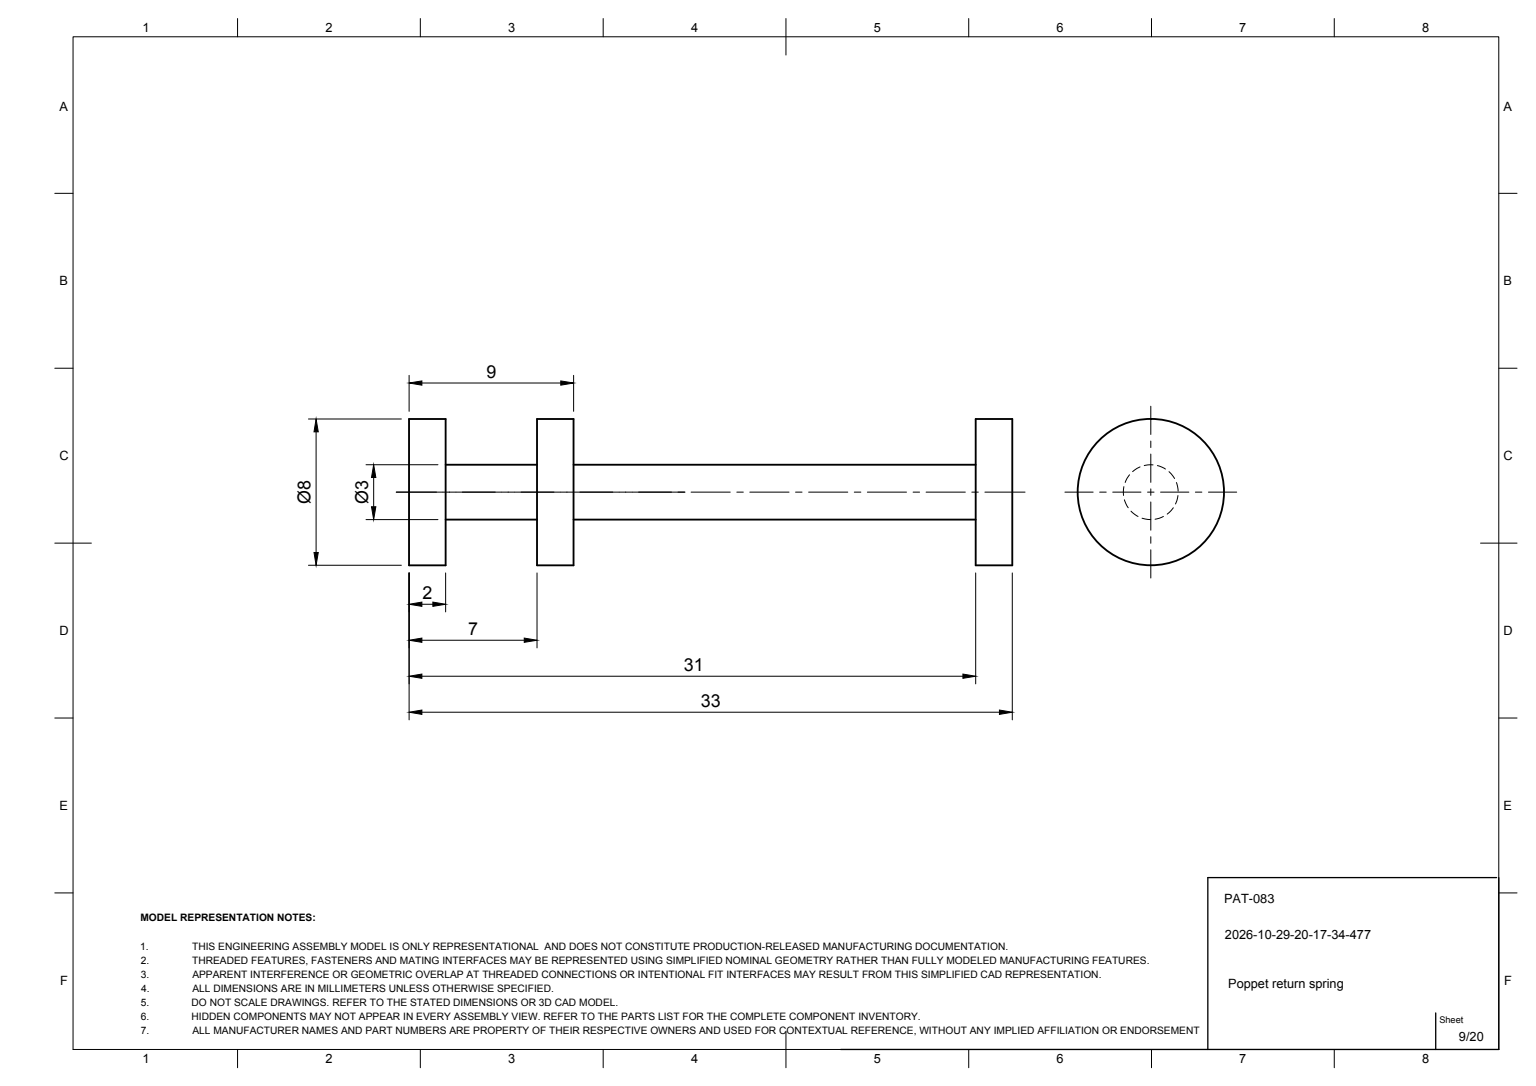
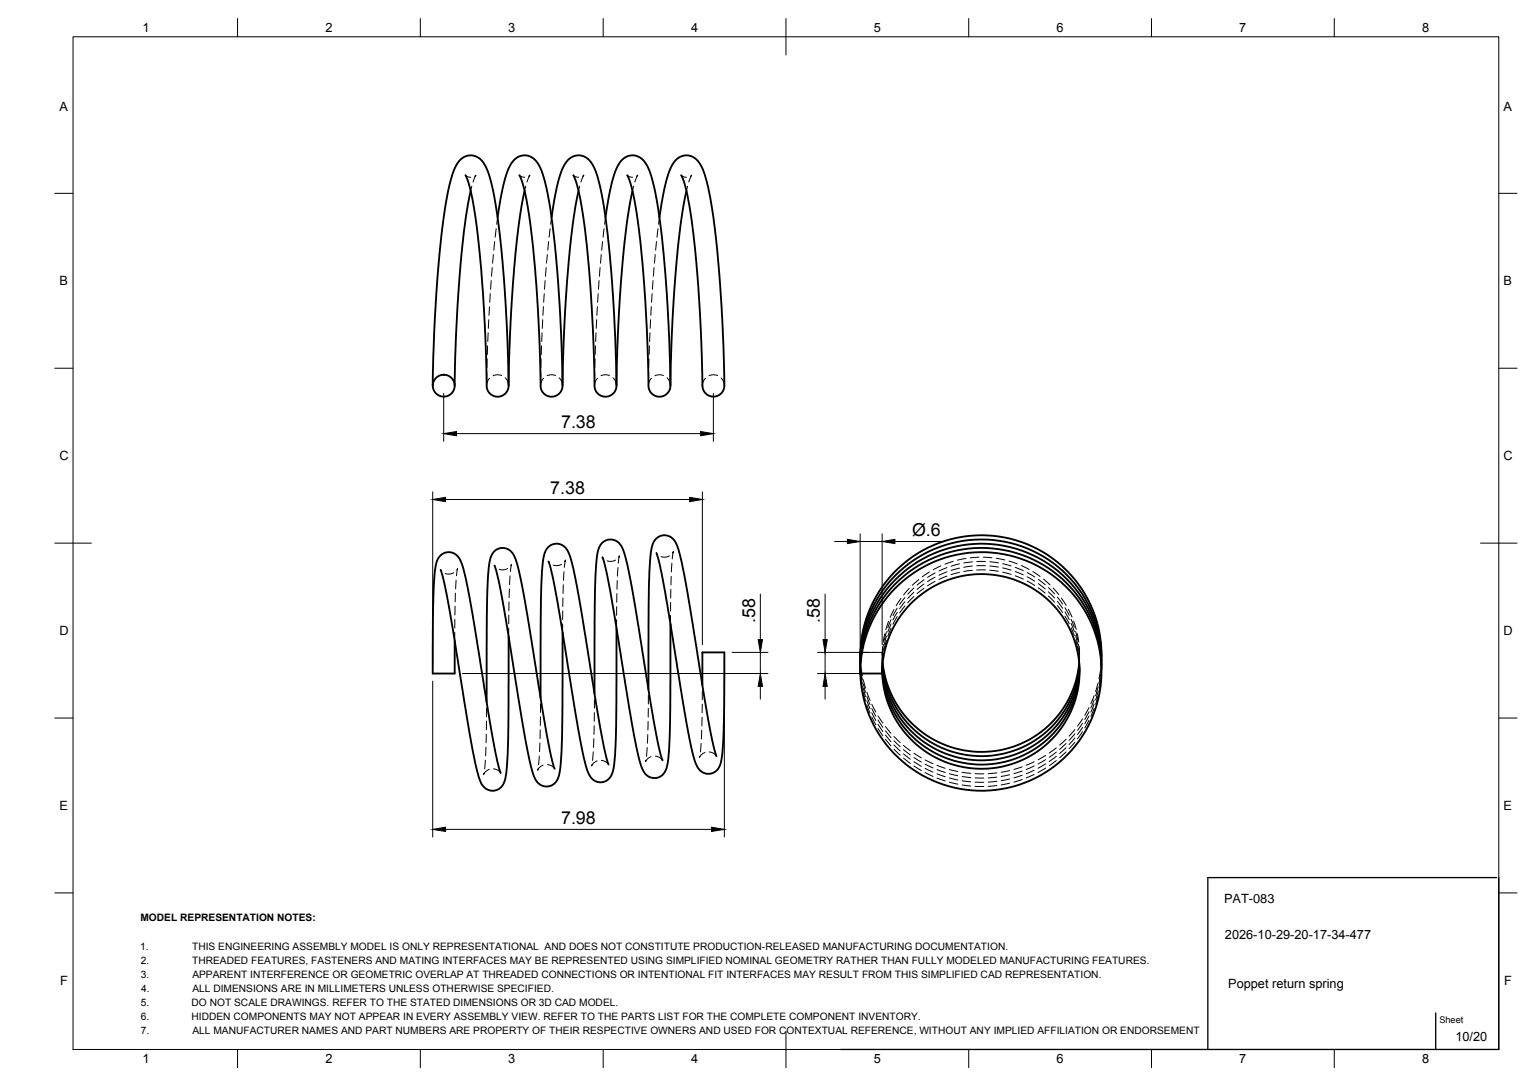
ISO-10303-21;
HEADER;
/* Generated by software containing ST-Developer
 * from STEP Tools, Inc. (www.steptools.com) 
 */

FILE_DESCRIPTION(
/* description */ ('PAT-083'),
/* implementation_level */ '2;1');

FILE_NAME(
/* name */ 'Poppet return spring.step',
/* time_stamp */ '2026-10-29T20:18:00-07:00',
/* author */ (''),
/* organization */ (''),
/* preprocessor_version */ 'ST-DEVELOPER v20.2',
/* originating_system */ 'Autodesk Translation Framework v15.17.0.0',
/* authorisation */ '');

FILE_SCHEMA (('AUTOMOTIVE_DESIGN { 1 0 10303 214 3 1 1 }'));
ENDSEC;

DATA;
#10=MECHANICAL_DESIGN_GEOMETRIC_PRESENTATION_REPRESENTATION('',(#236),#8428);
#165=B_SPLINE_SURFACE_WITH_KNOTS('',3,3,((#6072,#6073,#6074,#6075,#6076,
#6077,#6078,#6079,#6080,#6081,#6082,#6083,#6084,#6085,#6086,#6087,#6088,
#6089,#6090,#6091,#6092,#6093,#6094,#6095,#6096,#6097,#6098,#6099,#6100,
#6101,#6102,#6103,#6104,#6105,#6106,#6107,#6108,#6109,#6110,#6111,#6112,
#6113,#6114,#6115,#6116,#6117,#6118,#6119,#6120,#6121,#6122,#6123,#6124,
#6125,#6126,#6127,#6128,#6129,#6130,#6131,#6132),(#6133,#6134,#6135,#6136,
#6137,#6138,#6139,#6140,#6141,#6142,#6143,#6144,#6145,#6146,#6147,#6148,
#6149,#6150,#6151,#6152,#6153,#6154,#6155,#6156,#6157,#6158,#6159,#6160,
#6161,#6162,#6163,#6164,#6165,#6166,#6167,#6168,#6169,#6170,#6171,#6172,
#6173,#6174,#6175,#6176,#6177,#6178,#6179,#6180,#6181,#6182,#6183,#6184,
#6185,#6186,#6187,#6188,#6189,#6190,#6191,#6192,#6193),(#6194,#6195,#6196,
#6197,#6198,#6199,#6200,#6201,#6202,#6203,#6204,#6205,#6206,#6207,#6208,
#6209,#6210,#6211,#6212,#6213,#6214,#6215,#6216,#6217,#6218,#6219,#6220,
#6221,#6222,#6223,#6224,#6225,#6226,#6227,#6228,#6229,#6230,#6231,#6232,
#6233,#6234,#6235,#6236,#6237,#6238,#6239,#6240,#6241,#6242,#6243,#6244,
#6245,#6246,#6247,#6248,#6249,#6250,#6251,#6252,#6253,#6254),(#6255,#6256,
#6257,#6258,#6259,#6260,#6261,#6262,#6263,#6264,#6265,#6266,#6267,#6268,
#6269,#6270,#6271,#6272,#6273,#6274,#6275,#6276,#6277,#6278,#6279,#6280,
#6281,#6282,#6283,#6284,#6285,#6286,#6287,#6288,#6289,#6290,#6291,#6292,
#6293,#6294,#6295,#6296,#6297,#6298,#6299,#6300,#6301,#6302,#6303,#6304,
#6305,#6306,#6307,#6308,#6309,#6310,#6311,#6312,#6313,#6314,#6315),(#6316,
#6317,#6318,#6319,#6320,#6321,#6322,#6323,#6324,#6325,#6326,#6327,#6328,
#6329,#6330,#6331,#6332,#6333,#6334,#6335,#6336,#6337,#6338,#6339,#6340,
#6341,#6342,#6343,#6344,#6345,#6346,#6347,#6348,#6349,#6350,#6351,#6352,
#6353,#6354,#6355,#6356,#6357,#6358,#6359,#6360,#6361,#6362,#6363,#6364,
#6365,#6366,#6367,#6368,#6369,#6370,#6371,#6372,#6373,#6374,#6375,#6376),
(#6377,#6378,#6379,#6380,#6381,#6382,#6383,#6384,#6385,#6386,#6387,#6388,
#6389,#6390,#6391,#6392,#6393,#6394,#6395,#6396,#6397,#6398,#6399,#6400,
#6401,#6402,#6403,#6404,#6405,#6406,#6407,#6408,#6409,#6410,#6411,#6412,
#6413,#6414,#6415,#6416,#6417,#6418,#6419,#6420,#6421,#6422,#6423,#6424,
#6425,#6426,#6427,#6428,#6429,#6430,#6431,#6432,#6433,#6434,#6435,#6436,
#6437),(#6438,#6439,#6440,#6441,#6442,#6443,#6444,#6445,#6446,#6447,#6448,
#6449,#6450,#6451,#6452,#6453,#6454,#6455,#6456,#6457,#6458,#6459,#6460,
#6461,#6462,#6463,#6464,#6465,#6466,#6467,#6468,#6469,#6470,#6471,#6472,
#6473,#6474,#6475,#6476,#6477,#6478,#6479,#6480,#6481,#6482,#6483,#6484,
#6485,#6486,#6487,#6488,#6489,#6490,#6491,#6492,#6493,#6494,#6495,#6496,
#6497,#6498),(#6499,#6500,#6501,#6502,#6503,#6504,#6505,#6506,#6507,#6508,
#6509,#6510,#6511,#6512,#6513,#6514,#6515,#6516,#6517,#6518,#6519,#6520,
#6521,#6522,#6523,#6524,#6525,#6526,#6527,#6528,#6529,#6530,#6531,#6532,
#6533,#6534,#6535,#6536,#6537,#6538,#6539,#6540,#6541,#6542,#6543,#6544,
#6545,#6546,#6547,#6548,#6549,#6550,#6551,#6552,#6553,#6554,#6555,#6556,
#6557,#6558,#6559),(#6560,#6561,#6562,#6563,#6564,#6565,#6566,#6567,#6568,
#6569,#6570,#6571,#6572,#6573,#6574,#6575,#6576,#6577,#6578,#6579,#6580,
#6581,#6582,#6583,#6584,#6585,#6586,#6587,#6588,#6589,#6590,#6591,#6592,
#6593,#6594,#6595,#6596,#6597,#6598,#6599,#6600,#6601,#6602,#6603,#6604,
#6605,#6606,#6607,#6608,#6609,#6610,#6611,#6612,#6613,#6614,#6615,#6616,
#6617,#6618,#6619,#6620),(#6621,#6622,#6623,#6624,#6625,#6626,#6627,#6628,
#6629,#6630,#6631,#6632,#6633,#6634,#6635,#6636,#6637,#6638,#6639,#6640,
#6641,#6642,#6643,#6644,#6645,#6646,#6647,#6648,#6649,#6650,#6651,#6652,
#6653,#6654,#6655,#6656,#6657,#6658,#6659,#6660,#6661,#6662,#6663,#6664,
#6665,#6666,#6667,#6668,#6669,#6670,#6671,#6672,#6673,#6674,#6675,#6676,
#6677,#6678,#6679,#6680,#6681),(#6682,#6683,#6684,#6685,#6686,#6687,#6688,
#6689,#6690,#6691,#6692,#6693,#6694,#6695,#6696,#6697,#6698,#6699,#6700,
#6701,#6702,#6703,#6704,#6705,#6706,#6707,#6708,#6709,#6710,#6711,#6712,
#6713,#6714,#6715,#6716,#6717,#6718,#6719,#6720,#6721,#6722,#6723,#6724,
#6725,#6726,#6727,#6728,#6729,#6730,#6731,#6732,#6733,#6734,#6735,#6736,
#6737,#6738,#6739,#6740,#6741,#6742)),.UNSPECIFIED.,.T.,.F.,.F.,(4,1,1,
1,1,1,1,1,4),(4,1,1,1,1,1,1,1,1,1,1,1,1,1,1,1,1,1,1,1,1,1,1,1,1,1,1,1,1,
1,1,1,1,1,1,1,1,1,1,1,1,1,1,1,1,1,1,1,1,1,1,1,1,1,1,1,1,1,4),(-3.14159265358979,
-2.46839422782055,-2.24399475256414,-1.34639685153848,-0.448798950512828,
0.448798950512828,1.34639685153848,2.24399475256414,3.14159265358979),(0.,
0.0178571428571429,0.0357142857142857,0.0535714285714286,0.0714285714285714,
0.0892857142857143,0.107142857142857,0.125,0.129464285714286,0.133928571428571,
0.138392857142857,0.142857142857143,0.166666666666667,0.19047619047619,
0.214285714285714,0.232142857142857,0.25,0.267857142857143,0.285714285714286,
0.303571428571429,0.321428571428571,0.339285714285714,0.357142857142857,
0.375,0.392857142857143,0.410714285714286,0.428571428571429,0.446428571428571,
0.464285714285714,0.482142857142857,0.5,0.517857142857143,0.535714285714286,
0.553571428571429,0.571428571428571,0.589285714285714,0.607142857142857,
0.625,0.642857142857143,0.666666666666667,0.69047619047619,0.714285714285714,
0.726190476190476,0.738095238095238,0.761904761904762,0.767857142857143,
0.773809523809524,0.785714285714286,0.809523809523809,0.833333333333333,
0.857142857142857,0.875,0.892857142857143,0.910714285714286,0.928571428571429,
0.946428571428571,0.964285714285714,0.982142857142857,1.),.UNSPECIFIED.);
#176=B_SPLINE_CURVE_WITH_KNOTS('',3,(#6746,#6747,#6748,#6749,#6750,#6751,
#6752,#6753,#6754,#6755,#6756,#6757,#6758,#6759,#6760,#6761,#6762,#6763,
#6764,#6765,#6766,#6767,#6768,#6769,#6770,#6771,#6772,#6773,#6774,#6775,
#6776,#6777,#6778,#6779,#6780,#6781,#6782,#6783,#6784,#6785,#6786,#6787,
#6788,#6789,#6790,#6791,#6792,#6793,#6794,#6795,#6796,#6797,#6798,#6799,
#6800,#6801,#6802,#6803,#6804,#6805,#6806),.UNSPECIFIED.,.F.,.F.,(4,1,1,
1,1,1,1,1,1,1,1,1,1,1,1,1,1,1,1,1,1,1,1,1,1,1,1,1,1,1,1,1,1,1,1,1,1,1,1,
1,1,1,1,1,1,1,1,1,1,1,1,1,1,1,1,1,1,1,4),(0.,0.0178571428571429,0.0357142857142857,
0.0535714285714286,0.0714285714285714,0.0892857142857143,0.107142857142857,
0.125,0.129464285714286,0.133928571428571,0.138392857142857,0.142857142857143,
0.166666666666667,0.19047619047619,0.214285714285714,0.232142857142857,
0.25,0.267857142857143,0.285714285714286,0.303571428571429,0.321428571428571,
0.339285714285714,0.357142857142857,0.375,0.392857142857143,0.410714285714286,
0.428571428571429,0.446428571428571,0.464285714285714,0.482142857142857,
0.5,0.517857142857143,0.535714285714286,0.553571428571429,0.571428571428571,
0.589285714285714,0.607142857142857,0.625,0.642857142857143,0.666666666666667,
0.69047619047619,0.714285714285714,0.726190476190476,0.738095238095238,
0.761904761904762,0.767857142857143,0.773809523809524,0.785714285714286,
0.809523809523809,0.833333333333333,0.857142857142857,0.875,0.892857142857143,
0.910714285714286,0.928571428571429,0.946428571428571,0.964285714285714,
0.982142857142857,1.),.UNSPECIFIED.);
#188=SHAPE_REPRESENTATION_RELATIONSHIP('SRR','None',#8522,#212);
#212=ADVANCED_BREP_SHAPE_REPRESENTATION('',(#260),#8411);
#236=STYLED_ITEM('',(#8705),#260);
#260=MANIFOLD_SOLID_BREP('Body1',#3682);
#401=PLANE('',#4111);
#402=PLANE('',#4112);
#571=FACE_OUTER_BOUND('',#833,.T.);
#572=FACE_OUTER_BOUND('',#834,.T.);
#573=FACE_OUTER_BOUND('',#835,.T.);
#833=EDGE_LOOP('',(#2738,#2739,#2740,#2741));
#834=EDGE_LOOP('',(#2742));
#835=EDGE_LOOP('',(#2743));
#1588=CIRCLE('',#4109,0.03);
#1589=CIRCLE('',#4110,0.03);
#1801=VERTEX_POINT('',#6743);
#1802=VERTEX_POINT('',#6745);
#2145=EDGE_CURVE('',#1801,#1801,#1588,.T.);
#2146=EDGE_CURVE('',#1801,#1802,#176,.T.);
#2147=EDGE_CURVE('',#1802,#1802,#1589,.T.);
#2738=ORIENTED_EDGE('',*,*,#2145,.T.);
#2739=ORIENTED_EDGE('',*,*,#2146,.T.);
#2740=ORIENTED_EDGE('',*,*,#2147,.F.);
#2741=ORIENTED_EDGE('',*,*,#2146,.F.);
#2742=ORIENTED_EDGE('',*,*,#2147,.T.);
#2743=ORIENTED_EDGE('',*,*,#2145,.F.);
#3518=ADVANCED_FACE('',(#571),#165,.T.);
#3519=ADVANCED_FACE('',(#572),#401,.T.);
#3520=ADVANCED_FACE('',(#573),#402,.F.);
#3682=CLOSED_SHELL('',(#3518,#3519,#3520));
#4108=AXIS2_PLACEMENT_3D('',#6071,#4793,#4794);
#4109=AXIS2_PLACEMENT_3D('',#6744,#4795,#4796);
#4110=AXIS2_PLACEMENT_3D('',#6807,#4797,#4798);
#4111=AXIS2_PLACEMENT_3D('',#6808,#4799,#4800);
#4112=AXIS2_PLACEMENT_3D('',#6809,#4801,#4802);
#4793=DIRECTION('axis',(0.,0.,1.));
#4794=DIRECTION('refdir',(1.,0.,0.));
#4795=DIRECTION('center_axis',(-0.000134706207972677,0.996949949346912,
0.0780434516883255));
#4796=DIRECTION('ref_axis',(1.0545100428422E-5,-0.0780434509759074,0.99694995844755));
#4797=DIRECTION('center_axis',(0.000134706099743608,0.996949949299701,0.0780434522915993));
#4798=DIRECTION('ref_axis',(-0.630738728235735,0.0606460551105772,-0.77362181503826));
#4799=DIRECTION('center_axis',(0.000134706099743608,0.996949949299701,0.0780434522915993));
#4800=DIRECTION('ref_axis',(-0.630738728235735,0.0606460551105772,-0.77362181503826));
#4801=DIRECTION('center_axis',(-0.000134706207972677,0.996949949346912,
0.0780434516883255));
#4802=DIRECTION('ref_axis',(1.0545100428422E-5,-0.0780434509759074,0.99694995844755));
#6071=CARTESIAN_POINT('',(0.,0.,0.));
#6072=CARTESIAN_POINT('Ctrl Pts',(0.299999683646987,0.00234130352927725,
1.40009150124657));
#6073=CARTESIAN_POINT('Ctrl Pts',(0.299992075807792,0.058646317336039,1.40449918252257));
#6074=CARTESIAN_POINT('Ctrl Pts',(0.267703823976176,0.170873854805974,1.41332597689034));
#6075=CARTESIAN_POINT('Ctrl Pts',(0.136388292868123,0.288427001435921,1.42662720914847));
#6076=CARTESIAN_POINT('Ctrl Pts',(-0.0380600582278086,0.318117946543192,
1.43998475699785));
#6077=CARTESIAN_POINT('Ctrl Pts',(-0.202303265104397,0.250195717548651,
1.45340015631867));
#6078=CARTESIAN_POINT('Ctrl Pts',(-0.305668184856449,0.104682534491432,
1.46687214536364));
#6079=CARTESIAN_POINT('Ctrl Pts',(-0.315820032591246,-0.0743007733969036,
1.48040059247731));
#6080=CARTESIAN_POINT('Ctrl Pts',(-0.250581817185145,-0.192431453073831,
1.49058865012208));
#6081=CARTESIAN_POINT('Ctrl Pts',(-0.184885616277594,-0.249388366415835,
1.49739790674125));
#6082=CARTESIAN_POINT('Ctrl Pts',(-0.148390241821198,-0.273082371347815,
1.50080595723938));
#6083=CARTESIAN_POINT('Ctrl Pts',(-0.108871032283292,-0.29139234917315,
1.50421741983629));
#6084=CARTESIAN_POINT('Ctrl Pts',(-0.0069453324122751,-0.322535646049005,
1.51256485573429));
#6085=CARTESIAN_POINT('Ctrl Pts',(0.173036139719135,-0.295879163364944,
1.52588654224678));
#6086=CARTESIAN_POINT('Ctrl Pts',(0.329381275573112,-0.0995231210697565,
1.54425036939462));
#6087=CARTESIAN_POINT('Ctrl Pts',(0.312519823715869,0.130664619012925,1.56116776183919));
#6088=CARTESIAN_POINT('Ctrl Pts',(0.175623409891217,0.283196568811908,1.57661184582646));
#6089=CARTESIAN_POINT('Ctrl Pts',(-0.00170640174969724,0.334465005486407,
1.59056005485894));
#6090=CARTESIAN_POINT('Ctrl Pts',(-0.180023541764348,0.283195393823563,
1.60455538622492));
#6091=CARTESIAN_POINT('Ctrl Pts',(-0.304003293840334,0.144546913461868,
1.61859632997908));
#6092=CARTESIAN_POINT('Ctrl Pts',(-0.335368767729676,-0.0394152680933303,
1.63268129545808));
#6093=CARTESIAN_POINT('Ctrl Pts',(-0.263809464751215,-0.212364713608931,
1.64680860320332));
#6094=CARTESIAN_POINT('Ctrl Pts',(-0.110777353802162,-0.321042679653587,
1.66097649136357));
#6095=CARTESIAN_POINT('Ctrl Pts',(0.0771377319574853,-0.331662145388596,
1.67518312328143));
#6096=CARTESIAN_POINT('Ctrl Pts',(0.242310499059917,-0.240422185372272,
1.68942658430208));
#6097=CARTESIAN_POINT('Ctrl Pts',(0.333965165875749,-0.0749639048060816,
1.70370489167579));
#6098=CARTESIAN_POINT('Ctrl Pts',(0.323334808639096,0.114391665751362,1.71801599173701));
#6099=CARTESIAN_POINT('Ctrl Pts',(0.213428807823085,0.269386973572793,1.73235777220482));
#6100=CARTESIAN_POINT('Ctrl Pts',(0.0375551957208218,0.342290293088701,
1.74672805867088));
#6101=CARTESIAN_POINT('Ctrl Pts',(-0.150552157108958,0.310435266995363,
1.76112462104241));
#6102=CARTESIAN_POINT('Ctrl Pts',(-0.292943546037226,0.183080826664645,
1.7755451807512));
#6103=CARTESIAN_POINT('Ctrl Pts',(-0.345971724616545,-0.000755050169826696,
1.78998741229651));
#6104=CARTESIAN_POINT('Ctrl Pts',(-0.292969625414991,-0.184869584225357,
1.80444894933381));
#6105=CARTESIAN_POINT('Ctrl Pts',(-0.149964130695888,-0.312702949838195,
1.81892738366057));
#6106=CARTESIAN_POINT('Ctrl Pts',(0.0393278383702601,-0.344893411306051,
1.83342028161105));
#6107=CARTESIAN_POINT('Ctrl Pts',(0.216880569645654,-0.271353329755712,
1.84792517694669));
#6108=CARTESIAN_POINT('Ctrl Pts',(0.32816306590606,-0.114557947655581,1.86243958044385));
#6109=CARTESIAN_POINT('Ctrl Pts',(0.338976565498085,0.077604733921516,1.87696098559129));
#6110=CARTESIAN_POINT('Ctrl Pts',(0.245857394029791,0.245901091257368,1.8914868739057));
#6111=CARTESIAN_POINT('Ctrl Pts',(0.0587650041824393,0.349754038023421,
1.90762891978624));
#6112=CARTESIAN_POINT('Ctrl Pts',(-0.181113967151586,0.314103429348402,
1.92538434383923));
#6113=CARTESIAN_POINT('Ctrl Pts',(-0.3457209249242,0.106820407791971,1.94474686926749));
#6114=CARTESIAN_POINT('Ctrl Pts',(-0.329429326627219,-0.112545408830404,
1.96087146849268));
#6115=CARTESIAN_POINT('Ctrl Pts',(-0.229624239431613,-0.246663510889421,
1.97376168226292));
#6116=CARTESIAN_POINT('Ctrl Pts',(-0.0883709022792632,-0.335964900532689,
1.98664460529397));
#6117=CARTESIAN_POINT('Ctrl Pts',(0.0650538569064664,-0.336061455964098,
1.99790631348129));
#6118=CARTESIAN_POINT('Ctrl Pts',(0.175154846512334,-0.280150232411291,
2.00754964965835));
#6119=CARTESIAN_POINT('Ctrl Pts',(0.240313024233827,-0.230169139256515,
2.01397587403001));
#6120=CARTESIAN_POINT('Ctrl Pts',(0.327278516892606,-0.113059531596934,
2.02521445394406));
#6121=CARTESIAN_POINT('Ctrl Pts',(0.344164783870684,0.104896799870906,2.04124691031968));
#6122=CARTESIAN_POINT('Ctrl Pts',(0.180057434020278,0.310325992459091,2.06044404323233));
#6123=CARTESIAN_POINT('Ctrl Pts',(-0.0568089689745267,0.345505318367412,
2.07799813231589));
#6124=CARTESIAN_POINT('Ctrl Pts',(-0.24141865243425,0.243028671458529,2.09391813720595));
#6125=CARTESIAN_POINT('Ctrl Pts',(-0.332978054716675,0.0773726024996246,
2.1082144881335));
#6126=CARTESIAN_POINT('Ctrl Pts',(-0.322327341410981,-0.111361257795146,
2.12247707319913));
#6127=CARTESIAN_POINT('Ctrl Pts',(-0.213201521733808,-0.265029708724835,
2.13670391728446));
#6128=CARTESIAN_POINT('Ctrl Pts',(-0.0395013579051905,-0.33691517309109,
2.15089294308459));
#6129=CARTESIAN_POINT('Ctrl Pts',(0.145288666887708,-0.305489063077451,
2.16504251556762));
#6130=CARTESIAN_POINT('Ctrl Pts',(0.284599775362727,-0.18083938172608,2.17915024381374));
#6131=CARTESIAN_POINT('Ctrl Pts',(0.318914082780001,-0.0616119635988021,
2.18852795857496));
#6132=CARTESIAN_POINT('Ctrl Pts',(0.318922161847072,-0.0018193816533177,
2.19320865445115));
#6133=CARTESIAN_POINT('Ctrl Pts',(0.293267699450747,0.00234039391484394,
1.40009150124657));
#6134=CARTESIAN_POINT('Ctrl Pts',(0.293260260783866,0.0573933768638441,
1.404401170772));
#6135=CARTESIAN_POINT('Ctrl Pts',(0.261685961222457,0.167106937147775,1.41303112442804));
#6136=CARTESIAN_POINT('Ctrl Pts',(0.133284398422381,0.282057446849938,1.42603808763138));
#6137=CARTESIAN_POINT('Ctrl Pts',(-0.0373291122578389,0.311099769178308,
1.43910259661189));
#6138=CARTESIAN_POINT('Ctrl Pts',(-0.198000217206654,0.244664129919692,
1.45222664056713));
#6139=CARTESIAN_POINT('Ctrl Pts',(-0.299150297118565,0.10228514235472,1.46540970339088));
#6140=CARTESIAN_POINT('Ctrl Pts',(-0.309098158415524,-0.072901218291685,
1.47865182929301));
#6141=CARTESIAN_POINT('Ctrl Pts',(-0.245229011903188,-0.188573983871875,
1.48862820905086));
#6142=CARTESIAN_POINT('Ctrl Pts',(-0.180890303179359,-0.244355141625382,
1.49529690715063));
#6143=CARTESIAN_POINT('Ctrl Pts',(-0.145145442776525,-0.267562223220666,
1.49863493300563));
#6144=CARTESIAN_POINT('Ctrl Pts',(-0.106434830287264,-0.285497864023997,
1.50197663435114));
#6145=CARTESIAN_POINT('Ctrl Pts',(-0.00658463218961376,-0.31600740949559,
1.51015421506047));
#6146=CARTESIAN_POINT('Ctrl Pts',(0.169803335212638,-0.289904551356884,
1.52321054336867));
#6147=CARTESIAN_POINT('Ctrl Pts',(0.323140342136514,-0.0973784285380068,
1.54121822441294));
#6148=CARTESIAN_POINT('Ctrl Pts',(0.306625599321007,0.128498402162331,1.55781889560626));
#6149=CARTESIAN_POINT('Ctrl Pts',(0.172221287437576,0.278283700657156,1.57298361049915));
#6150=CARTESIAN_POINT('Ctrl Pts',(-0.00199515167689712,0.328668835140418,
1.58668730446444));
#6151=CARTESIAN_POINT('Ctrl Pts',(-0.177297430280052,0.278285030800204,
1.60044562410953));
#6152=CARTESIAN_POINT('Ctrl Pts',(-0.299269202723749,0.141909876792653,
1.61425746251936));
#6153=CARTESIAN_POINT('Ctrl Pts',(-0.330162486971795,-0.0391685498718976,
1.62812169321704));
#6154=CARTESIAN_POINT('Ctrl Pts',(-0.259693749447613,-0.209534410414459,
1.64203704930538));
#6155=CARTESIAN_POINT('Ctrl Pts',(-0.108859663184327,-0.316676626843527,
1.65600218178666));
#6156=CARTESIAN_POINT('Ctrl Pts',(0.076505205414545,-0.327173117244501,
1.6700156352621));
#6157=CARTESIAN_POINT('Ctrl Pts',(0.239569384718494,-0.237122125019053,
1.68407584770812));
#6158=CARTESIAN_POINT('Ctrl Pts',(0.330138826176287,-0.0736687244436319,
1.69818173535813));
#6159=CARTESIAN_POINT('Ctrl Pts',(0.319651197590554,0.113548934374436,1.71233030884879));
#6160=CARTESIAN_POINT('Ctrl Pts',(0.210918141794392,0.266931928573215,1.72652079296202));
#6161=CARTESIAN_POINT('Ctrl Pts',(0.0367565960986196,0.33914953789685,1.74075114688302));
#6162=CARTESIAN_POINT('Ctrl Pts',(-0.149685558776009,0.307602531834638,
1.75501873521155));
#6163=CARTESIAN_POINT('Ctrl Pts',(-0.290952593298896,0.181283052059042,
1.76932343108276));
#6164=CARTESIAN_POINT('Ctrl Pts',(-0.343624299509979,-0.00122470576221222,
1.78366073529875));
#6165=CARTESIAN_POINT('Ctrl Pts',(-0.290980868645007,-0.184182288319934,
1.79802970310735));
#6166=CARTESIAN_POINT('Ctrl Pts',(-0.148771903912068,-0.311336659778199,
1.81242794870657));
#6167=CARTESIAN_POINT('Ctrl Pts',(0.03964924936428,-0.343404204343566,1.82685321116496));
#6168=CARTESIAN_POINT('Ctrl Pts',(0.216555130910507,-0.270158948781549,
1.84130317466462));
#6169=CARTESIAN_POINT('Ctrl Pts',(0.327545313208071,-0.113818423308632,
1.85577536070366));
#6170=CARTESIAN_POINT('Ctrl Pts',(0.338363125822719,0.0779740906565071,
1.87026757403339));
#6171=CARTESIAN_POINT('Ctrl Pts',(0.245361396637451,0.246111297670799,1.88477684497455));
#6172=CARTESIAN_POINT('Ctrl Pts',(0.0583067834553886,0.349974365607058,
1.90091574842115));
#6173=CARTESIAN_POINT('Ctrl Pts',(-0.181787851399422,0.314354426222109,
1.91868303616071));
#6174=CARTESIAN_POINT('Ctrl Pts',(-0.346789882068873,0.106664965971596,
1.93808521951499));
#6175=CARTESIAN_POINT('Ctrl Pts',(-0.330496339658479,-0.113422069416505,
1.9542610714215));
#6176=CARTESIAN_POINT('Ctrl Pts',(-0.230283779721878,-0.248105619725249,
1.96720310592885));
#6177=CARTESIAN_POINT('Ctrl Pts',(-0.0883522547555857,-0.337843644550113,
1.98014846800894));
#6178=CARTESIAN_POINT('Ctrl Pts',(0.0659064686942833,-0.337971037882213,
1.99146805063414));
#6179=CARTESIAN_POINT('Ctrl Pts',(0.176715751168689,-0.281702711275593,
2.00117298579014));
#6180=CARTESIAN_POINT('Ctrl Pts',(0.242310061646865,-0.231388071089323,
2.00764183259477));
#6181=CARTESIAN_POINT('Ctrl Pts',(0.329896261130398,-0.113455911595648,
2.01895911802151));
#6182=CARTESIAN_POINT('Ctrl Pts',(0.346963705804559,0.106219379641946,2.03511657263834));
#6183=CARTESIAN_POINT('Ctrl Pts',(0.181421017200114,0.313529381253331,2.05448291591772));
#6184=CARTESIAN_POINT('Ctrl Pts',(-0.0578316111487914,0.349111887104915,
2.07221137618884));
#6185=CARTESIAN_POINT('Ctrl Pts',(-0.244497621198263,0.245521434385232,
2.08830552097745));
#6186=CARTESIAN_POINT('Ctrl Pts',(-0.337158982464816,0.0779154827919484,
2.1027691197373));
#6187=CARTESIAN_POINT('Ctrl Pts',(-0.326396740207177,-0.113196561520307,
2.11720948839641));
#6188=CARTESIAN_POINT('Ctrl Pts',(-0.215834447915981,-0.268925810611374,
2.1316241607543));
#6189=CARTESIAN_POINT('Ctrl Pts',(-0.0397023314431912,-0.341839636870502,
2.14601087914839));
#6190=CARTESIAN_POINT('Ctrl Pts',(0.147810528969888,-0.309966423960966,
2.16036733775139));
#6191=CARTESIAN_POINT('Ctrl Pts',(0.289279140671208,-0.183404826055055,
2.17469136125443));
#6192=CARTESIAN_POINT('Ctrl Pts',(0.32413793905981,-0.0622550446484658,
2.18421850306274));
#6193=CARTESIAN_POINT('Ctrl Pts',(0.324146149699815,-0.00148870109147552,
2.18897542715673));
#6194=CARTESIAN_POINT('Ctrl Pts',(0.284351574566012,0.00209289635755192,
1.4032377180594));
#6195=CARTESIAN_POINT('Ctrl Pts',(0.284344357328317,0.0555070994772719,
1.40741910026758));
#6196=CARTESIAN_POINT('Ctrl Pts',(0.253735841667482,0.161879987588016,1.41578500995075));
#6197=CARTESIAN_POINT('Ctrl Pts',(0.129255560771724,0.273321780593359,1.42839424570576));
#6198=CARTESIAN_POINT('Ctrl Pts',(-0.0361050419550946,0.301460299900524,
1.44105512584986));
#6199=CARTESIAN_POINT('Ctrl Pts',(-0.19180454726181,0.237074994443535,1.45377239878429));
#6200=CARTESIAN_POINT('Ctrl Pts',(-0.289812564223684,0.0991093413318229,
1.46654521640033));
#6201=CARTESIAN_POINT('Ctrl Pts',(-0.299447123537825,-0.070638578082909,
1.47937536902017));
#6202=CARTESIAN_POINT('Ctrl Pts',(-0.23755772335888,-0.182718163461684,
1.4890408587334));
#6203=CARTESIAN_POINT('Ctrl Pts',(-0.175208552710509,-0.236773567523899,
1.49550315164272));
#6204=CARTESIAN_POINT('Ctrl Pts',(-0.140568379573528,-0.259263236852212,
1.49873794667775));
#6205=CARTESIAN_POINT('Ctrl Pts',(-0.103053036763,-0.276644990895967,1.50197640326238));
#6206=CARTESIAN_POINT('Ctrl Pts',(-0.00628337548740407,-0.306213143561888,
1.50990159030283));
#6207=CARTESIAN_POINT('Ctrl Pts',(0.16466851405336,-0.280921166762252,1.52255426313202));
#6208=CARTESIAN_POINT('Ctrl Pts',(0.313343496448229,-0.094270090403481,
1.54001286072801));
#6209=CARTESIAN_POINT('Ctrl Pts',(0.297341035202232,0.124810650260335,1.55611362339848));
#6210=CARTESIAN_POINT('Ctrl Pts',(0.166930423314896,0.270157693737924,1.57082805896355));
#6211=CARTESIAN_POINT('Ctrl Pts',(-0.0021871479333846,0.319077064365966,
1.5841307898054));
#6212=CARTESIAN_POINT('Ctrl Pts',(-0.172445457813514,0.270153484695753,
1.5974930126463));
#6213=CARTESIAN_POINT('Ctrl Pts',(-0.290977247976819,0.137641678545292,
1.61091447749511));
#6214=CARTESIAN_POINT('Ctrl Pts',(-0.321026877647783,-0.038416870033602,
1.62439476923727));
#6215=CARTESIAN_POINT('Ctrl Pts',(-0.252480754699545,-0.204171031652774,
1.63793338359126));
#6216=CARTESIAN_POINT('Ctrl Pts',(-0.105644078858064,-0.30849214717115,
1.65152969033013));
#6217=CARTESIAN_POINT('Ctrl Pts',(0.0749472165069855,-0.318734659244124,
1.6651829598536));
#6218=CARTESIAN_POINT('Ctrl Pts',(0.233943323856699,-0.230950878459999,
1.67889234706262));
#6219=CARTESIAN_POINT('Ctrl Pts',(0.322332463437095,-0.0714702251109403,
1.69265670983326));
#6220=CARTESIAN_POINT('Ctrl Pts',(0.312110574480096,0.111369019946347,1.70647544116127));
#6221=CARTESIAN_POINT('Ctrl Pts',(0.205845454912002,0.261304060772099,1.72034700838273));
#6222=CARTESIAN_POINT('Ctrl Pts',(0.0354650074486262,0.331979400056782,
1.73427018684545));
#6223=CARTESIAN_POINT('Ctrl Pts',(-0.14711797487682,0.301106817491115,1.74824389266385));
#6224=CARTESIAN_POINT('Ctrl Pts',(-0.28560490328058,0.177309272695843,1.76226588379689));
#6225=CARTESIAN_POINT('Ctrl Pts',(-0.337309662661643,-0.00176488184415049,
1.77633558452815));
#6226=CARTESIAN_POINT('Ctrl Pts',(-0.285626419421087,-0.181478411719522,
1.79045084345521));
#6227=CARTESIAN_POINT('Ctrl Pts',(-0.145813563718198,-0.306526186142243,
1.80460998723798));
#6228=CARTESIAN_POINT('Ctrl Pts',(0.0396526632860302,-0.338118913343718,
1.81881118880055));
#6229=CARTESIAN_POINT('Ctrl Pts',(0.213993052827738,-0.265966707712057,
1.83305253571127));
#6230=CARTESIAN_POINT('Ctrl Pts',(0.323513667978463,-0.111746358162693,
1.84733208863259));
#6231=CARTESIAN_POINT('Ctrl Pts',(0.334229113099525,0.0776825567486598,
1.86164769315016));
#6232=CARTESIAN_POINT('Ctrl Pts',(0.242289928018038,0.243955698081078,1.87599744953428));
#6233=CARTESIAN_POINT('Ctrl Pts',(0.0571271931439024,0.346811227773582,
1.89197656081854));
#6234=CARTESIAN_POINT('Ctrl Pts',(-0.180921437098845,0.311556741369201,
1.90959711440866));
#6235=CARTESIAN_POINT('Ctrl Pts',(-0.344833685733874,0.105378317315944,
1.92886497432744));
#6236=CARTESIAN_POINT('Ctrl Pts',(-0.328686048836367,-0.11353363448047,
1.94495640357339));
#6237=CARTESIAN_POINT('Ctrl Pts',(-0.228894216428349,-0.247673192303685,
1.95784757972856));
#6238=CARTESIAN_POINT('Ctrl Pts',(-0.0874628865303489,-0.337117355536019,
1.97074826183704));
#6239=CARTESIAN_POINT('Ctrl Pts',(0.0665148567815164,-0.337289314963655,
1.98205225693581));
#6240=CARTESIAN_POINT('Ctrl Pts',(0.177201780714138,-0.281087394194614,
1.9917465206046));
#6241=CARTESIAN_POINT('Ctrl Pts',(0.24275024614819,-0.230808651930823,1.99821132889996));
#6242=CARTESIAN_POINT('Ctrl Pts',(0.330344232191523,-0.112890571889901,
2.009529543392));
#6243=CARTESIAN_POINT('Ctrl Pts',(0.347492403924234,0.10704864474084,2.02570982435864));
#6244=CARTESIAN_POINT('Ctrl Pts',(0.181535655882207,0.3150304141917,2.04513839975171));
#6245=CARTESIAN_POINT('Ctrl Pts',(-0.0588091737727422,0.350847169159054,
2.06295250484409));
#6246=CARTESIAN_POINT('Ctrl Pts',(-0.246611289832875,0.246670966545805,
2.07914587119244));
#6247=CARTESIAN_POINT('Ctrl Pts',(-0.339969156119851,0.0778684416628693,
2.09371690120608));
#6248=CARTESIAN_POINT('Ctrl Pts',(-0.329145769048135,-0.114860699832476,
2.10828205463687));
#6249=CARTESIAN_POINT('Ctrl Pts',(-0.217536412770799,-0.272112506388316,
2.12283904951299));
#6250=CARTESIAN_POINT('Ctrl Pts',(-0.0394980503574506,-0.345849044433683,
2.13738466058146));
#6251=CARTESIAN_POINT('Ctrl Pts',(0.150291350431643,-0.313616322822559,
2.15191771714466));
#6252=CARTESIAN_POINT('Ctrl Pts',(0.293659717677233,-0.185414557532162,
2.16643262471795));
#6253=CARTESIAN_POINT('Ctrl Pts',(0.329066204710721,-0.0625058077220191,
2.17610149040741));
#6254=CARTESIAN_POINT('Ctrl Pts',(0.329074534271164,-0.000859342736721239,
2.18092731235806));
#6255=CARTESIAN_POINT('Ctrl Pts',(0.271492587378726,0.00109723241378548,
1.41593442625805));
#6256=CARTESIAN_POINT('Ctrl Pts',(0.271485694290624,0.052112430132334,1.41992800900624));
#6257=CARTESIAN_POINT('Ctrl Pts',(0.242249559139038,0.153586730774769,1.42791007606117));
#6258=CARTESIAN_POINT('Ctrl Pts',(0.123659626324257,0.259706097017051,1.43992072996988));
#6259=CARTESIAN_POINT('Ctrl Pts',(-0.0335930623853517,0.286428140373609,
1.45196090010097));
#6260=CARTESIAN_POINT('Ctrl Pts',(-0.18141482672022,0.225267890136344,1.4640363624814));
#6261=CARTESIAN_POINT('Ctrl Pts',(-0.274318874126518,0.094438252948025,
1.47614773226753));
#6262=CARTESIAN_POINT('Ctrl Pts',(-0.283417169160825,-0.0663035653041664,
1.48829769185157));
#6263=CARTESIAN_POINT('Ctrl Pts',(-0.224864636858723,-0.172308199765865,
1.49744065450877));
#6264=CARTESIAN_POINT('Ctrl Pts',(-0.16593170165895,-0.223401513993078,
1.50354898148737));
#6265=CARTESIAN_POINT('Ctrl Pts',(-0.133197290901991,-0.244653576577957,
1.50660582486713));
#6266=CARTESIAN_POINT('Ctrl Pts',(-0.097754906384767,-0.261074677072147,
1.50966538240655));
#6267=CARTESIAN_POINT('Ctrl Pts',(-0.00635215241037408,-0.289001855159658,
1.51715100459395));
#6268=CARTESIAN_POINT('Ctrl Pts',(0.155004993833741,-0.265095701696411,
1.52909474424491));
#6269=CARTESIAN_POINT('Ctrl Pts',(0.295165120037499,-0.0890774075493339,
1.54555712282203));
#6270=CARTESIAN_POINT('Ctrl Pts',(0.280063643211613,0.11733841973294,1.56072753588602));
#6271=CARTESIAN_POINT('Ctrl Pts',(0.157246215363437,0.254211665897086,1.57458501593487));
#6272=CARTESIAN_POINT('Ctrl Pts',(-0.00197270028535737,0.300263721233418,
1.5871091434798));
#6273=CARTESIAN_POINT('Ctrl Pts',(-0.162235754907892,0.254210796053949,
1.59968706600409));
#6274=CARTESIAN_POINT('Ctrl Pts',(-0.273804433807857,0.129485742602018,
1.61231997991121));
#6275=CARTESIAN_POINT('Ctrl Pts',(-0.302094559974484,-0.0362384831563508,
1.62500901828759));
#6276=CARTESIAN_POINT('Ctrl Pts',(-0.237566582128313,-0.192294748298478,
1.63775518726396));
#6277=CARTESIAN_POINT('Ctrl Pts',(-0.0992882607141231,-0.290547628373896,
1.65055939320127));
#6278=CARTESIAN_POINT('Ctrl Pts',(0.0708532123640876,-0.300210016777284,
1.66342242123036));
#6279=CARTESIAN_POINT('Ctrl Pts',(0.220734377664724,-0.217475815836061,
1.67634494789799));
#6280=CARTESIAN_POINT('Ctrl Pts',(0.304120921236133,-0.0670576746065354,
1.6893276806875));
#6281=CARTESIAN_POINT('Ctrl Pts',(0.294493037088311,0.105526319670907,1.70237071363371));
#6282=CARTESIAN_POINT('Ctrl Pts',(0.194123591577484,0.247183982583743,1.71547466227991));
#6283=CARTESIAN_POINT('Ctrl Pts',(0.0330240595431114,0.314036071305745,
1.72863970901699));
#6284=CARTESIAN_POINT('Ctrl Pts',(-0.139805002589633,0.284842603775967,
1.74186572143678));
#6285=CARTESIAN_POINT('Ctrl Pts',(-0.271061350072721,0.167547140942527,
1.75515329680073));
#6286=CARTESIAN_POINT('Ctrl Pts',(-0.320149825119423,-0.0023451892674139,
1.76850151258264));
#6287=CARTESIAN_POINT('Ctrl Pts',(-0.271083065196151,-0.173086876640925,
1.78191051150415));
#6288=CARTESIAN_POINT('Ctrl Pts',(-0.138097485184967,-0.292077909506515,
1.79537986457642));
#6289=CARTESIAN_POINT('Ctrl Pts',(0.0385983399591338,-0.32221636504151,
1.80890908708627));
#6290=CARTESIAN_POINT('Ctrl Pts',(0.204974200986741,-0.253404878031692,
1.82249757886881));
#6291=CARTESIAN_POINT('Ctrl Pts',(0.30968647607717,-0.106029489164137,1.83614458498297));
#6292=CARTESIAN_POINT('Ctrl Pts',(0.319991027068231,0.0753271207673322,
1.84984935113891));
#6293=CARTESIAN_POINT('Ctrl Pts',(0.231853242034047,0.234821776128565,1.86361075588294));
#6294=CARTESIAN_POINT('Ctrl Pts',(0.0539694368211627,0.333696079427026,
1.87896342144752));
#6295=CARTESIAN_POINT('Ctrl Pts',(-0.175267053549315,0.299865670659702,
1.89592802781899));
#6296=CARTESIAN_POINT('Ctrl Pts',(-0.333627242296529,0.100875417751075,
1.91453010909236));
#6297=CARTESIAN_POINT('Ctrl Pts',(-0.318103980909791,-0.111059428495346,
1.9301070109208));
#6298=CARTESIAN_POINT('Ctrl Pts',(-0.221308531106851,-0.241211547793202,
1.94261179799545));
#6299=CARTESIAN_POINT('Ctrl Pts',(-0.0839111034095029,-0.328129409655272,
1.95514599042185));
#6300=CARTESIAN_POINT('Ctrl Pts',(0.0659787415594033,-0.328371864806453,
1.96614735699824));
#6301=CARTESIAN_POINT('Ctrl Pts',(0.173954717379698,-0.273553446450119,
1.97560349817015));
#6302=CARTESIAN_POINT('Ctrl Pts',(0.237941925838186,-0.224474378223391,
1.98191395714428));
#6303=CARTESIAN_POINT('Ctrl Pts',(0.323555514713298,-0.10925931253578,1.99297373967346));
#6304=CARTESIAN_POINT('Ctrl Pts',(0.340469789748638,0.106136096135639,2.00881942885412));
#6305=CARTESIAN_POINT('Ctrl Pts',(0.177559260022394,0.310550581792306,2.02790293557778));
#6306=CARTESIAN_POINT('Ctrl Pts',(-0.0592704015937349,0.345982341429199,
2.0454553049926));
#6307=CARTESIAN_POINT('Ctrl Pts',(-0.244890194023234,0.243100762578732,
2.06145549117311));
#6308=CARTESIAN_POINT('Ctrl Pts',(-0.337416126210674,0.0759330719099003,
2.07588653464397));
#6309=CARTESIAN_POINT('Ctrl Pts',(-0.326737063233083,-0.115421783027243,
2.09034610228147));
#6310=CARTESIAN_POINT('Ctrl Pts',(-0.215715969562994,-0.271959300347246,
2.10483205671323));
#6311=CARTESIAN_POINT('Ctrl Pts',(-0.0381314606062155,-0.345579124738108,
2.1193413423825));
#6312=CARTESIAN_POINT('Ctrl Pts',(0.151660986646548,-0.313406934885558,
2.13387292093976));
#6313=CARTESIAN_POINT('Ctrl Pts',(0.295411443757773,-0.184948656073821,
2.14842109049688));
#6314=CARTESIAN_POINT('Ctrl Pts',(0.331011968991107,-0.0614504945185775,
2.15813557967852));
#6315=CARTESIAN_POINT('Ctrl Pts',(0.331020345667048,0.000544668811153922,
2.16298869850864));
#6316=CARTESIAN_POINT('Ctrl Pts',(0.266533420052219,-0.000598446861652248,
1.43758697109781));
#6317=CARTESIAN_POINT('Ctrl Pts',(0.26652665376501,0.0494783075173114,1.44150709042139));
#6318=CARTESIAN_POINT('Ctrl Pts',(0.237828564223823,0.148934102677714,1.44933094401217));
#6319=CARTESIAN_POINT('Ctrl Pts',(0.121941169632728,0.252533932703974,1.46106241271628));
#6320=CARTESIAN_POINT('Ctrl Pts',(-0.031148631117057,0.278475984569276,
1.47278278595574));
#6321=CARTESIAN_POINT('Ctrl Pts',(-0.174537915324736,0.219070557052679,
1.4844981379325));
#6322=CARTESIAN_POINT('Ctrl Pts',(-0.264320512406116,0.0925130070182829,
1.49620987741958));
#6323=CARTESIAN_POINT('Ctrl Pts',(-0.273019793758845,-0.0624384219482381,
1.50792159815808));
#6324=CARTESIAN_POINT('Ctrl Pts',(-0.216708588582917,-0.164278737895499,
1.51670721227717));
#6325=CARTESIAN_POINT('Ctrl Pts',(-0.160180892291219,-0.213283628024979,
1.52256612937649));
#6326=CARTESIAN_POINT('Ctrl Pts',(-0.128805227872014,-0.233652238038377,
1.5254959752123));
#6327=CARTESIAN_POINT('Ctrl Pts',(-0.0948602906438099,-0.249378490854682,
1.5284262570081));
#6328=CARTESIAN_POINT('Ctrl Pts',(-0.0073795378077737,-0.27610445683934,
1.53559033771115));
#6329=CARTESIAN_POINT('Ctrl Pts',(0.146673956766819,-0.253167685233027,
1.54699409155007));
#6330=CARTESIAN_POINT('Ctrl Pts',(0.279896500835626,-0.0856285728439146,
1.56265532418908));
#6331=CARTESIAN_POINT('Ctrl Pts',(0.265458901440563,0.110056712248341,1.57703752301133));
#6332=CARTESIAN_POINT('Ctrl Pts',(0.149308581978497,0.239404593439139,1.59013780265147));
#6333=CARTESIAN_POINT('Ctrl Pts',(-0.000879246359104834,0.282794954861585,
1.60195050522868));
#6334=CARTESIAN_POINT('Ctrl Pts',(-0.15169922660277,0.239404889893613,1.61378836786326));
#6335=CARTESIAN_POINT('Ctrl Pts',(-0.256457774506062,0.122226885907837,
1.62565404553147));
#6336=CARTESIAN_POINT('Ctrl Pts',(-0.282939238014729,-0.0331463294577391,
1.63755013589437));
#6337=CARTESIAN_POINT('Ctrl Pts',(-0.222513907990111,-0.179181116194557,
1.6494791816529));
#6338=CARTESIAN_POINT('Ctrl Pts',(-0.0932867834705937,-0.270960294371653,
1.66144366426743));
#6339=CARTESIAN_POINT('Ctrl Pts',(0.0654677283059359,-0.279944637602497,
1.67344599120345));
#6340=CARTESIAN_POINT('Ctrl Pts',(0.205124760040014,-0.202822617250478,
1.68548851375222));
#6341=CARTESIAN_POINT('Ctrl Pts',(0.282720976254736,-0.0627985050799433,
1.69757329221837));
#6342=CARTESIAN_POINT('Ctrl Pts',(0.273746547884209,0.0976912909106923,
1.70970294432419));
#6343=CARTESIAN_POINT('Ctrl Pts',(0.180471658752939,0.229304408207884,1.72187920671603));
#6344=CARTESIAN_POINT('Ctrl Pts',(0.0308764741788442,0.291367908294201,
1.73410415425347));
#6345=CARTESIAN_POINT('Ctrl Pts',(-0.129523158214965,0.264262077447812,
1.74637987496184));
#6346=CARTESIAN_POINT('Ctrl Pts',(-0.251291518773948,0.155437729951258,
1.75870764348809));
#6347=CARTESIAN_POINT('Ctrl Pts',(-0.296820627951342,-0.00215178387272073,
1.77108984108917));
#6348=CARTESIAN_POINT('Ctrl Pts',(-0.251309762852418,-0.160519102576093,
1.78352773391814));
#6349=CARTESIAN_POINT('Ctrl Pts',(-0.127952255814083,-0.270899775685238,
1.79602286205806));
#6350=CARTESIAN_POINT('Ctrl Pts',(0.0359923471661857,-0.298870254746358,
1.8085766053069));
#6351=CARTESIAN_POINT('Ctrl Pts',(0.190426644024177,-0.235008880970683,
1.82119023321984));
#6352=CARTESIAN_POINT('Ctrl Pts',(0.287682855256994,-0.0981507875079271,
1.83386492806554));
#6353=CARTESIAN_POINT('Ctrl Pts',(0.297276612211721,0.0703845270426061,
1.84660167249208));
#6354=CARTESIAN_POINT('Ctrl Pts',(0.215320379043628,0.218732235998905,1.85940151393512));
#6355=CARTESIAN_POINT('Ctrl Pts',(0.0497410880640545,0.310798493864736,
1.87369422624341));
#6356=CARTESIAN_POINT('Ctrl Pts',(-0.163934573054978,0.279322056893055,
1.88950895549613));
#6357=CARTESIAN_POINT('Ctrl Pts',(-0.311842090402094,0.093597039791909,
1.90687638344953));
#6358=CARTESIAN_POINT('Ctrl Pts',(-0.297389946716595,-0.104635041214907,
1.92144675642255));
#6359=CARTESIAN_POINT('Ctrl Pts',(-0.206725724713414,-0.226570099612231,
1.9331617974391));
#6360=CARTESIAN_POINT('Ctrl Pts',(-0.0778995181755873,-0.308087964657102,
1.94491517743614));
#6361=CARTESIAN_POINT('Ctrl Pts',(0.0629117092812275,-0.308372369450851,
1.95525227591192));
#6362=CARTESIAN_POINT('Ctrl Pts',(0.164490964977537,-0.256807355278177,
1.96414796506574));
#6363=CARTESIAN_POINT('Ctrl Pts',(0.224722944339505,-0.21060994633766,1.97008821946209));
#6364=CARTESIAN_POINT('Ctrl Pts',(0.305401073256525,-0.10206812301548,1.98050932509365));
#6365=CARTESIAN_POINT('Ctrl Pts',(0.321462965061058,0.101261332430962,1.99546946518584));
#6366=CARTESIAN_POINT('Ctrl Pts',(0.167353833457747,0.294860683101063,2.01353713913069));
#6367=CARTESIAN_POINT('Ctrl Pts',(-0.0574805364540771,0.328622162338068,
2.03020314733791));
#6368=CARTESIAN_POINT('Ctrl Pts',(-0.234210607295154,0.230747071427096,
2.04543515185281));
#6369=CARTESIAN_POINT('Ctrl Pts',(-0.322547239746861,0.0712703181694491,
2.05920591331795));
#6370=CARTESIAN_POINT('Ctrl Pts',(-0.312395670542285,-0.111759879847481,
2.07303733322864));
#6371=CARTESIAN_POINT('Ctrl Pts',(-0.205992467238026,-0.26189561908817,
2.08692864153008));
#6372=CARTESIAN_POINT('Ctrl Pts',(-0.035301754120549,-0.33272882463994,
2.10087770204531));
#6373=CARTESIAN_POINT('Ctrl Pts',(0.147640705043926,-0.301785489794866,
2.11488504909042));
#6374=CARTESIAN_POINT('Ctrl Pts',(0.286610389683,-0.177698918117886,2.12894498467352));
#6375=CARTESIAN_POINT('Ctrl Pts',(0.321161806690122,-0.0580367709741704,
2.13835992180599));
#6376=CARTESIAN_POINT('Ctrl Pts',(0.32116993299807,0.00210543722720802,
2.14306798720062));
#6377=CARTESIAN_POINT('Ctrl Pts',(0.285097284651427,-0.00241889983639149,
1.46087401350103));
#6378=CARTESIAN_POINT('Ctrl Pts',(0.285090059199041,0.0510560995578562,
1.46506015497633));
#6379=CARTESIAN_POINT('Ctrl Pts',(0.254405463959297,0.157243204973338,1.47341492833332));
#6380=CARTESIAN_POINT('Ctrl Pts',(0.131112493365165,0.267329197540611,1.48588887820255));
#6381=CARTESIAN_POINT('Ctrl Pts',(-0.0310790590612892,0.294737110561081,
1.49830621261202));
#6382=CARTESIAN_POINT('Ctrl Pts',(-0.182346981068028,0.231966474128732,
1.51066809926437));
#6383=CARTESIAN_POINT('Ctrl Pts',(-0.276622840120502,0.0989160846808463,
1.52297638590209));
#6384=CARTESIAN_POINT('Ctrl Pts',(-0.28562935546202,-0.0632450379079678,
1.53523274919662));
#6385=CARTESIAN_POINT('Ctrl Pts',(-0.226890031412833,-0.169325517012616,
1.54438751719497));
#6386=CARTESIAN_POINT('Ctrl Pts',(-0.168150306427595,-0.220243786261342,
1.55047565341104));
#6387=CARTESIAN_POINT('Ctrl Pts',(-0.135581939101061,-0.241384906042715,
1.55351674869088));
#6388=CARTESIAN_POINT('Ctrl Pts',(-0.100387654468105,-0.257688371292987,
1.55655490244068));
#6389=CARTESIAN_POINT('Ctrl Pts',(-0.0097824441123277,-0.285365009758757,
1.56397439181196));
#6390=CARTESIAN_POINT('Ctrl Pts',(0.149173126959868,-0.261514184936789,
1.5757425298963));
#6391=CARTESIAN_POINT('Ctrl Pts',(0.285602172828371,-0.0895278583518576,
1.59180512762946));
#6392=CARTESIAN_POINT('Ctrl Pts',(0.270659165239267,0.10990564271393,1.60646359224198));
#6393=CARTESIAN_POINT('Ctrl Pts',(0.152845360024874,0.240914998182156,1.61974140254765));
#6394=CARTESIAN_POINT('Ctrl Pts',(0.00132058495251339,0.284586289092117,
1.63165684771419));
#6395=CARTESIAN_POINT('Ctrl Pts',(-0.150052838385872,0.240923309697256,
1.6435401615279));
#6396=CARTESIAN_POINT('Ctrl Pts',(-0.254628743279724,0.123790276438128,
1.65539393682687));
#6397=CARTESIAN_POINT('Ctrl Pts',(-0.280852713971101,-0.0307010402102851,
1.66722078080952));
#6398=CARTESIAN_POINT('Ctrl Pts',(-0.220968814531156,-0.175151607286856,
1.67902337392248));
#6399=CARTESIAN_POINT('Ctrl Pts',(-0.0936586927728087,-0.265441896093515,
1.69080443492152));
#6400=CARTESIAN_POINT('Ctrl Pts',(0.0619320971189879,-0.274144025980544,
1.70256672698207));
#6401=CARTESIAN_POINT('Ctrl Pts',(0.198109144806248,-0.198827325563695,
1.71431302884181));
#6402=CARTESIAN_POINT('Ctrl Pts',(0.273365251138184,-0.0628212764942574,
1.72604644031572));
#6403=CARTESIAN_POINT('Ctrl Pts',(0.264591572289594,0.0922867316427776,
1.73776923268641));
#6404=CARTESIAN_POINT('Ctrl Pts',(0.174764652560144,0.218869799124979,1.74948474865086));
#6405=CARTESIAN_POINT('Ctrl Pts',(0.0314157170558157,0.278239262102867,
1.76119576873161));
#6406=CARTESIAN_POINT('Ctrl Pts',(-0.121576817067625,0.252291826805016,
1.77290499016194));
#6407=CARTESIAN_POINT('Ctrl Pts',(-0.237194160915694,0.148844679759727,
1.7846159414541));
#6408=CARTESIAN_POINT('Ctrl Pts',(-0.280189871842215,-0.000283120495965188,
1.79633073217163));
#6409=CARTESIAN_POINT('Ctrl Pts',(-0.237216648905561,-0.149519446584567,
1.80805264345696));
#6410=CARTESIAN_POINT('Ctrl Pts',(-0.121334725719892,-0.253103788167418,
1.8197845112682));
#6411=CARTESIAN_POINT('Ctrl Pts',(0.032065824366413,-0.279197448292019,
1.83152919415975));
#6412=CARTESIAN_POINT('Ctrl Pts',(0.176032876548686,-0.219585186162864,
1.8432895314691));
#6413=CARTESIAN_POINT('Ctrl Pts',(0.266363672526068,-0.0923525264685545,
1.85506830270555));
#6414=CARTESIAN_POINT('Ctrl Pts',(0.275185263312216,0.0638000977606677,
1.86686833472312));
#6415=CARTESIAN_POINT('Ctrl Pts',(0.19942055667018,0.200817401186163,1.87869222140788));
#6416=CARTESIAN_POINT('Ctrl Pts',(0.0468336660220393,0.285581780166665,
1.89185969859235));
#6417=CARTESIAN_POINT('Ctrl Pts',(-0.149427870647855,0.256552776774109,
1.90638482005989));
#6418=CARTESIAN_POINT('Ctrl Pts',(-0.284785839872206,0.0863936580923987,
1.92228945474259));
#6419=CARTESIAN_POINT('Ctrl Pts',(-0.271505592195012,-0.0946541618773216,
1.93559641358745));
#6420=CARTESIAN_POINT('Ctrl Pts',(-0.18883448665128,-0.205814296251183,
1.94627666316605));
#6421=CARTESIAN_POINT('Ctrl Pts',(-0.0714878972225447,-0.280048650077599,
1.95698178449418));
#6422=CARTESIAN_POINT('Ctrl Pts',(0.056557422971355,-0.280266379011788,
1.96638001843711));
#6423=CARTESIAN_POINT('Ctrl Pts',(0.148842638659517,-0.233416525658896,
1.97446193547615));
#6424=CARTESIAN_POINT('Ctrl Pts',(0.203544042920288,-0.191460234672681,
1.97985660168861));
#6425=CARTESIAN_POINT('Ctrl Pts',(0.276766158498589,-0.0929323996780253,
1.9893151942404));
#6426=CARTESIAN_POINT('Ctrl Pts',(0.291296648239029,0.0914545316801896,
2.002880442837));
#6427=CARTESIAN_POINT('Ctrl Pts',(0.151649974014536,0.266828988428087,2.01924800893444));
#6428=CARTESIAN_POINT('Ctrl Pts',(-0.051938403746315,0.297387291798137,
2.03433788910338));
#6429=CARTESIAN_POINT('Ctrl Pts',(-0.211943418815992,0.20877346918723,2.04812762550537));
#6430=CARTESIAN_POINT('Ctrl Pts',(-0.291927406141446,0.0643829424248649,
2.06059498063548));
#6431=CARTESIAN_POINT('Ctrl Pts',(-0.282742302054825,-0.101374482622084,
2.0731204043778));
#6432=CARTESIAN_POINT('Ctrl Pts',(-0.18634967584022,-0.237409536214224,
2.08570530126253));
#6433=CARTESIAN_POINT('Ctrl Pts',(-0.0316120397930279,-0.301638279150675,
2.09835073112393));
#6434=CARTESIAN_POINT('Ctrl Pts',(0.13437413324299,-0.27359223176401,2.11105823551128));
#6435=CARTESIAN_POINT('Ctrl Pts',(0.260600324022261,-0.160901490961837,
2.1238278967204));
#6436=CARTESIAN_POINT('Ctrl Pts',(0.292024278813734,-0.0521464631533842,
2.13238426955925));
#6437=CARTESIAN_POINT('Ctrl Pts',(0.292031677431713,0.00261016504483008,
2.13667073981128));
#6438=CARTESIAN_POINT('Ctrl Pts',(0.314888635514893,-0.00241091183326431,
1.46082339350253));
#6439=CARTESIAN_POINT('Ctrl Pts',(0.31488066604922,0.0565704708297952,1.46544058686453));
#6440=CARTESIAN_POINT('Ctrl Pts',(0.281007406696283,0.173862408081188,1.47466873695446));
#6441=CARTESIAN_POINT('Ctrl Pts',(0.144847554197953,0.295426491012178,1.48844337668646));
#6442=CARTESIAN_POINT('Ctrl Pts',(-0.0342851373916114,0.325706577815792,
1.50215841582855));
#6443=CARTESIAN_POINT('Ctrl Pts',(-0.201331441874071,0.256378388746261,
1.51580959638849));
#6444=CARTESIAN_POINT('Ctrl Pts',(-0.305399495530267,0.109489858454975,
1.52939761607679));
#6445=CARTESIAN_POINT('Ctrl Pts',(-0.315320196692728,-0.0694407339097994,
1.54292114176174));
#6446=CARTESIAN_POINT('Ctrl Pts',(-0.250539306529347,-0.18639704075144,
1.55301514961419));
#6447=CARTESIAN_POINT('Ctrl Pts',(-0.18580905138686,-0.242506716265914,
1.55972411928833));
#6448=CARTESIAN_POINT('Ctrl Pts',(-0.149927816391745,-0.265797847575212,
1.56307451809262));
#6449=CARTESIAN_POINT('Ctrl Pts',(-0.111163875464346,-0.283754347820401,
1.566420820712));
#6450=CARTESIAN_POINT('Ctrl Pts',(-0.011394113389426,-0.314229695144002,
1.57459065039502));
#6451=CARTESIAN_POINT('Ctrl Pts',(0.163474807395259,-0.28793328486503,1.5875374009987));
#6452=CARTESIAN_POINT('Ctrl Pts',(0.313213210997328,-0.0990169221446236,
1.60517584236345));
#6453=CARTESIAN_POINT('Ctrl Pts',(0.296744609610656,0.119492548342282,1.62123688662316));
#6454=CARTESIAN_POINT('Ctrl Pts',(0.167905869182534,0.262670401766488,1.63575254694344));
#6455=CARTESIAN_POINT('Ctrl Pts',(0.00259435741764641,0.310260621883403,
1.64875115909385));
#6456=CARTESIAN_POINT('Ctrl Pts',(-0.162138978273715,0.262681198120579,
1.66168469519045));
#6457=CARTESIAN_POINT('Ctrl Pts',(-0.275621710656057,0.135476363579829,
1.67455370237198));
#6458=CARTESIAN_POINT('Ctrl Pts',(-0.303947788371616,-0.0318025544323174,
1.68735884399675));
#6459=CARTESIAN_POINT('Ctrl Pts',(-0.239232326675737,-0.187720156696059,
1.70010091014339));
#6460=CARTESIAN_POINT('Ctrl Pts',(-0.102168915306409,-0.284835237870766,
1.71278081298448));
#6461=CARTESIAN_POINT('Ctrl Pts',(0.0647507693491276,-0.294091793930313,
1.72539958234459));
#6462=CARTESIAN_POINT('Ctrl Pts',(0.210302405961457,-0.213496390348748,
1.7379583760209));
#6463=CARTESIAN_POINT('Ctrl Pts',(0.290399378819606,-0.0685648846902543,
1.75045830668886));
#6464=CARTESIAN_POINT('Ctrl Pts',(0.280997576102868,0.0960562826133116,
1.76290109090414));
#6465=CARTESIAN_POINT('Ctrl Pts',(0.185951839499003,0.229833807773724,1.77528794274805));
#6466=CARTESIAN_POINT('Ctrl Pts',(0.0349645157607975,0.292265615993788,
1.78762050889942));
#6467=CARTESIAN_POINT('Ctrl Pts',(-0.125462570041385,0.26495688981232,1.79990064341502));
#6468=CARTESIAN_POINT('Ctrl Pts',(-0.246125469550108,0.156864561640384,
1.81212970168938));
#6469=CARTESIAN_POINT('Ctrl Pts',(-0.290730578144321,0.00178869821857768,
1.82431014291597));
#6470=CARTESIAN_POINT('Ctrl Pts',(-0.246152133523863,-0.152651683052016,
1.83644367698913));
#6471=CARTESIAN_POINT('Ctrl Pts',(-0.126682433121871,-0.25930391813005,
1.84853242569022));
#6472=CARTESIAN_POINT('Ctrl Pts',(0.0306642005710787,-0.285962041058737,
1.86057855192037));
#6473=CARTESIAN_POINT('Ctrl Pts',(0.177586179060693,-0.225011410333218,
1.87258430463161));
#6474=CARTESIAN_POINT('Ctrl Pts',(0.26927399222783,-0.095683591155606,1.88455203531386));
#6475=CARTESIAN_POINT('Ctrl Pts',(0.278084925824305,0.0622130540219098,
1.8964840977736));
#6476=CARTESIAN_POINT('Ctrl Pts',(0.201753576721663,0.200038156901172,1.90838307166345));
#6477=CARTESIAN_POINT('Ctrl Pts',(0.0488818383881024,0.284820769561344,
1.92156992514232));
#6478=CARTESIAN_POINT('Ctrl Pts',(-0.146535093892137,0.25567223899667,1.93603617489917));
#6479=CARTESIAN_POINT('Ctrl Pts',(-0.280249802687413,0.0871596115803118,
1.9517731940105));
#6480=CARTESIAN_POINT('Ctrl Pts',(-0.266987101998673,-0.090825328261591,
1.96485665128121));
#6481=CARTESIAN_POINT('Ctrl Pts',(-0.186064361045936,-0.199562543379855,
1.97530826657453));
#6482=CARTESIAN_POINT('Ctrl Pts',(-0.0715738890859495,-0.27194086119468,
1.98575016408737));
#6483=CARTESIAN_POINT('Ctrl Pts',(0.0527681653931571,-0.272020816451964,
1.99487777982029));
#6484=CARTESIAN_POINT('Ctrl Pts',(0.142020233979434,-0.226699224433259,
2.00269503679117));
#6485=CARTESIAN_POINT('Ctrl Pts',(0.194849199560625,-0.186175829667411,
2.00790531695633));
#6486=CARTESIAN_POINT('Ctrl Pts',(0.26538453361425,-0.0912003750099694,
2.01702045742602));
#6487=CARTESIAN_POINT('Ctrl Pts',(0.279140342627061,0.0857273504720853,
2.03003586593044));
#6488=CARTESIAN_POINT('Ctrl Pts',(0.145738477869324,0.25287900544541,2.04565135075897));
#6489=CARTESIAN_POINT('Ctrl Pts',(-0.0474301726531468,0.281679315861089,
2.05996861217462));
#6490=CARTESIAN_POINT('Ctrl Pts',(-0.198476529428579,0.197914796760607,
2.07299160637881));
#6491=CARTESIAN_POINT('Ctrl Pts',(-0.273651952890791,0.0620394523940554,
2.08472102715745));
#6492=CARTESIAN_POINT('Ctrl Pts',(-0.264962198551285,-0.0933233659048604,
2.09646205614446));
#6493=CARTESIAN_POINT('Ctrl Pts',(-0.174865697747918,-0.220344133944316,
2.1082173622539));
#6494=CARTESIAN_POINT('Ctrl Pts',(-0.0307882849390207,-0.28006808447709,
2.11999016920861));
#6495=CARTESIAN_POINT('Ctrl Pts',(0.123235668238189,-0.253987402111434,
2.13178230852711));
#6496=CARTESIAN_POINT('Ctrl Pts',(0.239978957267943,-0.14966309953415,2.14359862418644));
#6497=CARTESIAN_POINT('Ctrl Pts',(0.268938930763692,-0.0493657724660812,
2.15148951655109));
#6498=CARTESIAN_POINT('Ctrl Pts',(0.268945755514944,0.00114371023782948,
2.15544351083781));
#6499=CARTESIAN_POINT('Ctrl Pts',(0.33350426217158,-0.00059269602393798,
1.43762910263796));
#6500=CARTESIAN_POINT('Ctrl Pts',(0.33349582470557,0.0618523199636564,1.44251743689346));
#6501=CARTESIAN_POINT('Ctrl Pts',(0.29762198454481,0.186264933883794,1.45230507780882));
#6502=CARTESIAN_POINT('Ctrl Pts',(0.152822448193178,0.315652416567409,1.46695951175481));
#6503=CARTESIAN_POINT('Ctrl Pts',(-0.0383328670928585,0.348050441216263,
1.48159650359311));
#6504=CARTESIAN_POINT('Ctrl Pts',(-0.217170947159076,0.273915243990747,
1.49620901228621));
#6505=CARTESIAN_POINT('Ctrl Pts',(-0.328953907481535,0.116273487480008,
1.51079639226664));
#6506=CARTESIAN_POINT('Ctrl Pts',(-0.339710227550737,-0.0763447775316334,
1.52535497546158));
#6507=CARTESIAN_POINT('Ctrl Pts',(-0.269832110033659,-0.202616097899319,
1.53625099803897));
#6508=CARTESIAN_POINT('Ctrl Pts',(-0.199851822715115,-0.263279824833576,
1.54350421430842));
#6509=CARTESIAN_POINT('Ctrl Pts',(-0.161036601589138,-0.28847685119871,
1.54712869281073));
#6510=CARTESIAN_POINT('Ctrl Pts',(-0.119075517257528,-0.30791540642489,
1.55075099769877));
#6511=CARTESIAN_POINT('Ctrl Pts',(-0.0110145788198074,-0.340926517013328,
1.55960012258723));
#6512=CARTESIAN_POINT('Ctrl Pts',(0.178779397072994,-0.312500615344175,
1.57365122925557));
#6513=CARTESIAN_POINT('Ctrl Pts',(0.341888081512569,-0.106946886916083,
1.59285101394101));
#6514=CARTESIAN_POINT('Ctrl Pts',(0.324027764111286,0.131568208827147,1.6103821375933));
#6515=CARTESIAN_POINT('Ctrl Pts',(0.183128836209753,0.288235889823992,1.6262610920956));
#6516=CARTESIAN_POINT('Ctrl Pts',(0.00199318449518641,0.340425594849694,
1.64050492212001));
#6517=CARTESIAN_POINT('Ctrl Pts',(-0.178814710744046,0.288246874522815,
1.65469959848629));
#6518=CARTESIAN_POINT('Ctrl Pts',(-0.303564976297722,0.148465660357223,
1.66884320009202));
#6519=CARTESIAN_POINT('Ctrl Pts',(-0.334766024780997,-0.0356039414078766,
1.68293395112495));
#6520=CARTESIAN_POINT('Ctrl Pts',(-0.263501466362289,-0.207369781260881,
1.69697015402715));
#6521=CARTESIAN_POINT('Ctrl Pts',(-0.112393993862094,-0.314462369886333,
1.71095022654457));
#6522=CARTESIAN_POINT('Ctrl Pts',(0.0717736879435312,-0.324692465946504,
1.72487268877397));
#6523=CARTESIAN_POINT('Ctrl Pts',(0.232455731514219,-0.235732487197711,
1.73873617356272));
#6524=CARTESIAN_POINT('Ctrl Pts',(0.320912988717144,-0.075688900837101,
1.75253956750793));
#6525=CARTESIAN_POINT('Ctrl Pts',(0.310531286438101,0.106125972684126,1.76628140037764));
#6526=CARTESIAN_POINT('Ctrl Pts',(0.205561190534091,0.253868234028805,1.77996092667565));
#6527=CARTESIAN_POINT('Ctrl Pts',(0.0388485409594955,0.322793218532066,
1.79357721819808));
#6528=CARTESIAN_POINT('Ctrl Pts',(-0.138202688744248,0.292642348031099,
1.80712928930927));
#6529=CARTESIAN_POINT('Ctrl Pts',(-0.271275014593156,0.173407667511399,
1.82061706508718));
#6530=CARTESIAN_POINT('Ctrl Pts',(-0.320408925286595,0.00250707464856787,
1.83403929175697));
#6531=CARTESIAN_POINT('Ctrl Pts',(-0.271307561449736,-0.167502591654885,
1.84739594116571));
#6532=CARTESIAN_POINT('Ctrl Pts',(-0.139930069519496,-0.284741206103476,
1.86068668924461));
#6533=CARTESIAN_POINT('Ctrl Pts',(0.0328273431379415,-0.313971999555478,
1.87391139490108));
#6534=CARTESIAN_POINT('Ctrl Pts',(0.193850817302591,-0.247125271575551,
1.88707004452662));
#6535=CARTESIAN_POINT('Ctrl Pts',(0.294125420947596,-0.105604428080939,
1.90016271438992));
#6536=CARTESIAN_POINT('Ctrl Pts',(0.303692393078913,0.0667945151618661,
1.91318971435693));
#6537=CARTESIAN_POINT('Ctrl Pts',(0.220491612017706,0.216911798478523,1.92615123879903));
#6538=CARTESIAN_POINT('Ctrl Pts',(0.0543221488869225,0.308989602518454,
1.94048115461963));
#6539=CARTESIAN_POINT('Ctrl Pts',(-0.157372149186157,0.277269028654297,
1.95615139456308));
#6540=CARTESIAN_POINT('Ctrl Pts',(-0.301541028549258,0.0952925261463745,
1.97313495002146));
#6541=CARTESIAN_POINT('Ctrl Pts',(-0.287140150837315,-0.0959909714068033,
1.98719573515425));
#6542=CARTESIAN_POINT('Ctrl Pts',(-0.200435907040306,-0.212440976387684,
1.99839033332071));
#6543=CARTESIAN_POINT('Ctrl Pts',(-0.0780453719389616,-0.28977073304184,
2.00955053962068));
#6544=CARTESIAN_POINT('Ctrl Pts',(0.0543569638846216,-0.289744106383568,
2.01926770009008));
#6545=CARTESIAN_POINT('Ctrl Pts',(0.149101826267907,-0.241622389761838,
2.0275666737348));
#6546=CARTESIAN_POINT('Ctrl Pts',(0.205114290476602,-0.198654311142817,
2.03309084965727));
#6547=CARTESIAN_POINT('Ctrl Pts',(0.27973233129585,-0.0981224791338798,
2.04273613227868));
#6548=CARTESIAN_POINT('Ctrl Pts',(0.294054838307538,0.0883885612962322,
2.05645362185213));
#6549=CARTESIAN_POINT('Ctrl Pts',(0.154021552042581,0.263442571251684,2.07282008366875));
#6550=CARTESIAN_POINT('Ctrl Pts',(-0.0473319417941907,0.293245461580669,
2.08774066257839));
#6551=CARTESIAN_POINT('Ctrl Pts',(-0.203892531954146,0.206287815842515,
2.10124325457571));
#6552=CARTESIAN_POINT('Ctrl Pts',(-0.281404389454363,0.0659836006472725,
2.11334963792451));
#6553=CARTESIAN_POINT('Ctrl Pts',(-0.2723714341636,-0.0936469583069963,
2.12541249039876));
#6554=CARTESIAN_POINT('Ctrl Pts',(-0.180144499604908,-0.22349377921263,
2.13743356131539));
#6555=CARTESIAN_POINT('Ctrl Pts',(-0.033449858406456,-0.284188291922273,
2.14941608862722));
#6556=CARTESIAN_POINT('Ctrl Pts',(0.122562408333805,-0.257670230647596,
2.16136028851425));
#6557=CARTESIAN_POINT('Ctrl Pts',(0.240186761064639,-0.15240311537952,2.17327325875895));
#6558=CARTESIAN_POINT('Ctrl Pts',(0.269167385254141,-0.0517780507002695,
2.18118730964103));
#6559=CARTESIAN_POINT('Ctrl Pts',(0.269174221747938,-0.00118166228325439,
2.18514810709965));
#6560=CARTESIAN_POINT('Ctrl Pts',(0.326819743817693,0.00167503652268494,
1.40864888399464));
#6561=CARTESIAN_POINT('Ctrl Pts',(0.326811467432193,0.0629279084542433,
1.41344389457114));
#6562=CARTESIAN_POINT('Ctrl Pts',(0.291654883267632,0.185084755965569,1.42305190526743));
#6563=CARTESIAN_POINT('Ctrl Pts',(0.148979195665167,0.312728390774808,1.43749916035482));
#6564=CARTESIAN_POINT('Ctrl Pts',(-0.0401862647160889,0.344885051828254,
1.45198374992715));
#6565=CARTESIAN_POINT('Ctrl Pts',(-0.217915663488207,0.271323343912871,
1.46650201744433));
#6566=CARTESIAN_POINT('Ctrl Pts',(-0.329503050990644,0.11413535024708,1.48105194869708));
#6567=CARTESIAN_POINT('Ctrl Pts',(-0.340379991513863,-0.0787520881849125,
1.49563081925542));
#6568=CARTESIAN_POINT('Ctrl Pts',(-0.270194290476258,-0.205738111213707,
1.50658459018308));
#6569=CARTESIAN_POINT('Ctrl Pts',(-0.199665121692685,-0.266881734670431,
1.51389467077294));
#6570=CARTESIAN_POINT('Ctrl Pts',(-0.160508386513694,-0.292302289608028,
1.51755114629707));
#6571=CARTESIAN_POINT('Ctrl Pts',(-0.118134791271926,-0.311933522239942,
1.52120901254844));
#6572=CARTESIAN_POINT('Ctrl Pts',(-0.00891167038672465,-0.34530394763833,
1.53015375485378));
#6573=CARTESIAN_POINT('Ctrl Pts',(0.183545882213297,-0.316669327909261,
1.54439993961451));
#6574=CARTESIAN_POINT('Ctrl Pts',(0.349995676828839,-0.107322625109419,
1.56396823487425));
#6575=CARTESIAN_POINT('Ctrl Pts',(0.331923882036601,0.137035034007625,1.58192781905788));
#6576=CARTESIAN_POINT('Ctrl Pts',(0.187023028957292,0.298335739363874,1.59826723674814));
#6577=CARTESIAN_POINT('Ctrl Pts',(-4.07900050576479E-5,0.352333628668086,
1.61297947284543));
#6578=CARTESIAN_POINT('Ctrl Pts',(-0.187515823756079,0.298337661946181,
1.62769561588367));
#6579=CARTESIAN_POINT('Ctrl Pts',(-0.317396577254554,0.152955414784301,
1.64241275153056));
#6580=CARTESIAN_POINT('Ctrl Pts',(-0.350074819871636,-0.0392507736732478,
1.65712799589898));
#6581=CARTESIAN_POINT('Ctrl Pts',(-0.275476950657307,-0.219299124116455,
1.67183845174987));
#6582=CARTESIAN_POINT('Ctrl Pts',(-0.116616564764591,-0.331999825553172,
1.68654123824752));
#6583=CARTESIAN_POINT('Ctrl Pts',(0.0777212807640258,-0.342885743881358,
1.70123348729869));
#6584=CARTESIAN_POINT('Ctrl Pts',(0.247890378833861,-0.248774962677378,
1.71591238391807));
#6585=CARTESIAN_POINT('Ctrl Pts',(0.341922241756374,-0.078821833086168,
1.73057458398919));
#6586=CARTESIAN_POINT('Ctrl Pts',(0.330944684888561,0.114920758632994,1.74521844664416));
#6587=CARTESIAN_POINT('Ctrl Pts',(0.218814809338252,0.272877094249764,1.75984029215667));
#6588=CARTESIAN_POINT('Ctrl Pts',(0.0401314023515666,0.346836885301389,
1.77443759960673));
#6589=CARTESIAN_POINT('Ctrl Pts',(-0.150221108850721,0.314496168181013,
1.78900816640339));
#6590=CARTESIAN_POINT('Ctrl Pts',(-0.293718171085479,0.18601886476932,1.80354799050301));
#6591=CARTESIAN_POINT('Ctrl Pts',(-0.346887342757174,0.00132400703486514,
1.81805626188758));
#6592=CARTESIAN_POINT('Ctrl Pts',(-0.29374715104042,-0.182902252872154,
1.83252961218796));
#6593=CARTESIAN_POINT('Ctrl Pts',(-0.151100609616018,-0.310278813236866,
1.84696571621268));
#6594=CARTESIAN_POINT('Ctrl Pts',(0.036937675316398,-0.342153332252125,
1.86136221026647));
#6595=CARTESIAN_POINT('Ctrl Pts',(0.212600699807242,-0.269287017513481,
1.8757168020348));
#6596=CARTESIAN_POINT('Ctrl Pts',(0.322231809337099,-0.114646253272976,
1.89002735257157));
#6597=CARTESIAN_POINT('Ctrl Pts',(0.332752609394029,0.0741069817676853,
1.9042916032421));
#6598=CARTESIAN_POINT('Ctrl Pts',(0.241542314658912,0.238754649423423,1.91850785152287));
#6599=CARTESIAN_POINT('Ctrl Pts',(0.0590639411267381,0.339919964670031,
1.93424736852057));
#6600=CARTESIAN_POINT('Ctrl Pts',(-0.17381495037296,0.305089861920068,1.95148870566044));
#6601=CARTESIAN_POINT('Ctrl Pts',(-0.332680466671874,0.104668687805014,
1.97019858165979));
#6602=CARTESIAN_POINT('Ctrl Pts',(-0.316831768055502,-0.10629215319313,
1.98570712860886));
#6603=CARTESIAN_POINT('Ctrl Pts',(-0.221152704671616,-0.234803595695131,
1.99806246070239));
#6604=CARTESIAN_POINT('Ctrl Pts',(-0.0860643901141648,-0.320165941287256,
2.01038082890037));
#6605=CARTESIAN_POINT('Ctrl Pts',(0.0601723380717702,-0.320146023962333,
2.02111670840766));
#6606=CARTESIAN_POINT('Ctrl Pts',(0.164800899338872,-0.26700416951472,2.03028161334532));
#6607=CARTESIAN_POINT('Ctrl Pts',(0.226657697996288,-0.21955265481665,2.03638255025733));
#6608=CARTESIAN_POINT('Ctrl Pts',(0.309065692640364,-0.108527426828177,
2.04703540530036));
#6609=CARTESIAN_POINT('Ctrl Pts',(0.324864915209835,0.0974261798297048,
2.0621845157232));
#6610=CARTESIAN_POINT('Ctrl Pts',(0.170289646488671,0.290611127431389,2.08025095052217));
#6611=CARTESIAN_POINT('Ctrl Pts',(-0.0517408616129622,0.323427973004647,
2.09670599777649));
#6612=CARTESIAN_POINT('Ctrl Pts',(-0.224161216243688,0.227626661550434,
2.11157970065908));
#6613=CARTESIAN_POINT('Ctrl Pts',(-0.309409326351099,0.0732552725630971,
2.1249004530645));
#6614=CARTESIAN_POINT('Ctrl Pts',(-0.299447065361936,-0.102125940306812,
2.13815531539376));
#6615=CARTESIAN_POINT('Ctrl Pts',(-0.198240680027746,-0.244539701723245,
2.15134406230612));
#6616=CARTESIAN_POINT('Ctrl Pts',(-0.037581548944414,-0.310964665237426,
2.16446709692427));
#6617=CARTESIAN_POINT('Ctrl Pts',(0.13292631747297,-0.281926222953237,2.17752364320475));
#6618=CARTESIAN_POINT('Ctrl Pts',(0.261173528224478,-0.167098336597803,
2.19051601295533));
#6619=CARTESIAN_POINT('Ctrl Pts',(0.292688581739866,-0.0575687444849278,
2.1991314360511));
#6620=CARTESIAN_POINT('Ctrl Pts',(0.292696006824134,-0.00261624123410937,
2.20343323983651));
#6621=CARTESIAN_POINT('Ctrl Pts',(0.308975662575307,0.00234251634852165,
1.40009150124657));
#6622=CARTESIAN_POINT('Ctrl Pts',(0.308967831215322,0.0603017897770032,
1.40462868163228));
#6623=CARTESIAN_POINT('Ctrl Pts',(0.27571613946542,0.17587293159813,1.41371870232149));
#6624=CARTESIAN_POINT('Ctrl Pts',(0.14052829168136,0.296880373272056,1.42741147339166));
#6625=CARTESIAN_POINT('Ctrl Pts',(-0.0390206409894663,0.327438852492569,
1.44115991935023));
#6626=CARTESIAN_POINT('Ctrl Pts',(-0.208015130690645,0.257544971295796,
1.45496360199322));
#6627=CARTESIAN_POINT('Ctrl Pts',(-0.31433121628426,0.107867391812847,1.46882103730561));
#6628=CARTESIAN_POINT('Ctrl Pts',(-0.324760930696744,-0.0761651731846545,
1.48273114655387));
#6629=CARTESIAN_POINT('Ctrl Pts',(-0.25770578826527,-0.197572131035348,
1.49320208134784));
#6630=CARTESIAN_POINT('Ctrl Pts',(-0.190205012752425,-0.256093277277717,
1.5001983760536));
#6631=CARTESIAN_POINT('Ctrl Pts',(-0.152711571444389,-0.280435204755278,
1.50369961169923));
#6632=CARTESIAN_POINT('Ctrl Pts',(-0.112116765219087,-0.299243448878827,
1.50720391497013));
#6633=CARTESIAN_POINT('Ctrl Pts',(-0.00742947447965367,-0.331230533315626,
1.51577743597841));
#6634=CARTESIAN_POINT('Ctrl Pts',(0.177344946592297,-0.303843669093901,
1.52945317895053));
#6635=CARTESIAN_POINT('Ctrl Pts',(0.337703669147259,-0.102384061208339,
1.54829190470144));
#6636=CARTESIAN_POINT('Ctrl Pts',(0.320386176990543,0.133556219760536,1.5656314880469));
#6637=CARTESIAN_POINT('Ctrl Pts',(0.180166649314842,0.289758997557382,1.58144797134203));
#6638=CARTESIAN_POINT('Ctrl Pts',(-0.00132206741687621,0.342212241169513,
1.59572221082199));
#6639=CARTESIAN_POINT('Ctrl Pts',(-0.183671702176775,0.289762637032663,
1.61003353536495));
#6640=CARTESIAN_POINT('Ctrl Pts',(-0.310342042497228,0.14807517418719,1.62437994961569));
#6641=CARTESIAN_POINT('Ctrl Pts',(-0.342344710230546,-0.0397483446680867,
1.63875921097831));
#6642=CARTESIAN_POINT('Ctrl Pts',(-0.26932802481127,-0.216162780784306,
1.65316909672021));
#6643=CARTESIAN_POINT('Ctrl Pts',(-0.11335028157701,-0.32690499085044,1.66760727054012));
#6644=CARTESIAN_POINT('Ctrl Pts',(0.0779896409308878,-0.337694308008293,
1.68207139079433));
#6645=CARTESIAN_POINT('Ctrl Pts',(0.245996504618211,-0.244859320987887,
1.69655892082441));
#6646=CARTESIAN_POINT('Ctrl Pts',(0.339122881244892,-0.0766951990321318,
1.71106887668148));
#6647=CARTESIAN_POINT('Ctrl Pts',(0.328303231554949,0.115536603234434,1.72559559277298));
#6648=CARTESIAN_POINT('Ctrl Pts',(0.216819416451737,0.272714660222625,1.74013907788606));
#6649=CARTESIAN_POINT('Ctrl Pts',(0.038629327840624,0.34654572302245,1.75469616476247));
#6650=CARTESIAN_POINT('Ctrl Pts',(-0.151730517540076,0.314282626901279,
1.76926319982864));
#6651=CARTESIAN_POINT('Ctrl Pts',(-0.295660631610015,0.185509220768529,
1.78384089368189));
#6652=CARTESIAN_POINT('Ctrl Pts',(-0.349181464322731,-0.000132902452383927,
1.79842245055717));
#6653=CARTESIAN_POINT('Ctrl Pts',(-0.295691618391146,-0.185833876958624,
1.81300730099236));
#6654=CARTESIAN_POINT('Ctrl Pts',(-0.151591431305487,-0.314604885214695,
1.82759256023074));
#6655=CARTESIAN_POINT('Ctrl Pts',(0.0389096325415752,-0.346969520413954,
1.84217561365937));
#6656=CARTESIAN_POINT('Ctrl Pts',(0.217372400747471,-0.273018514558698,
1.85675384492571));
#6657=CARTESIAN_POINT('Ctrl Pts',(0.329077169033808,-0.115573796608772,
1.87132449448901));
#6658=CARTESIAN_POINT('Ctrl Pts',(0.339888552571612,0.0771370427329227,
1.88588525710813));
#6659=CARTESIAN_POINT('Ctrl Pts',(0.246588824585348,0.245699401156214,1.90043285415478));
#6660=CARTESIAN_POINT('Ctrl Pts',(0.059383764715569,0.349570705626663,1.91658113980667));
#6661=CARTESIAN_POINT('Ctrl Pts',(-0.18025714962302,0.313891514320666,1.93431457393113));
#6662=CARTESIAN_POINT('Ctrl Pts',(-0.344390369949343,0.107068479425964,
1.95362750530272));
#6663=CARTESIAN_POINT('Ctrl Pts',(-0.328107849431858,-0.111399267400055,
1.96968435665062));
#6664=CARTESIAN_POINT('Ctrl Pts',(-0.228819035002148,-0.244801895274471,
1.98250464766913));
#6665=CARTESIAN_POINT('Ctrl Pts',(-0.0883888817388162,-0.333562219825158,
1.99531159404308));
#6666=CARTESIAN_POINT('Ctrl Pts',(0.06390108694825,-0.333615078896201,2.00648565100655));
#6667=CARTESIAN_POINT('Ctrl Pts',(0.17311235742343,-0.278151693895792,2.01605104836969));
#6668=CARTESIAN_POINT('Ctrl Pts',(0.237719738978489,-0.228592221119887,
2.0224225577694));
#6669=CARTESIAN_POINT('Ctrl Pts',(0.323887551888167,-0.112533970996369,
2.03355824516288));
#6670=CARTESIAN_POINT('Ctrl Pts',(0.340546892843711,0.103204150446501,2.04942473071775));
#6671=CARTESIAN_POINT('Ctrl Pts',(0.178299428106273,0.30616933398131,2.06839251648277));
#6672=CARTESIAN_POINT('Ctrl Pts',(-0.0554521422788362,0.340822969043152,
2.08571206561153));
#6673=CARTESIAN_POINT('Ctrl Pts',(-0.237391185083363,0.23979008338321,2.10140096499742));
#6674=CARTESIAN_POINT('Ctrl Pts',(-0.327514552494945,0.0766773806508595,
2.11547453862722));
#6675=CARTESIAN_POINT('Ctrl Pts',(-0.317013490278782,-0.108949377210494,
2.12950042186005));
#6676=CARTESIAN_POINT('Ctrl Pts',(-0.209773689761217,-0.259921362839895,
2.14347676014655));
#6677=CARTESIAN_POINT('Ctrl Pts',(-0.0392672842831704,-0.330457204877932,
2.15740251507558));
#6678=CARTESIAN_POINT('Ctrl Pts',(0.1419314616349,-0.299620592696538,2.17127537907273));
#6679=CARTESIAN_POINT('Ctrl Pts',(0.278394560994794,-0.177472560454167,
2.18509599978749));
#6680=CARTESIAN_POINT('Ctrl Pts',(0.311948936733415,-0.0607866435023563,
2.1942713847311));
#6681=CARTESIAN_POINT('Ctrl Pts',(0.311956844710082,-0.00226028906910728,
2.19885295751038));
#6682=CARTESIAN_POINT('Ctrl Pts',(0.299999683646987,0.00234130352927725,
1.40009150124657));
#6683=CARTESIAN_POINT('Ctrl Pts',(0.299992075807792,0.058646317336039,1.40449918252257));
#6684=CARTESIAN_POINT('Ctrl Pts',(0.267703823976176,0.170873854805974,1.41332597689034));
#6685=CARTESIAN_POINT('Ctrl Pts',(0.136388292868123,0.288427001435921,1.42662720914847));
#6686=CARTESIAN_POINT('Ctrl Pts',(-0.0380600582278086,0.318117946543192,
1.43998475699785));
#6687=CARTESIAN_POINT('Ctrl Pts',(-0.202303265104397,0.250195717548651,
1.45340015631867));
#6688=CARTESIAN_POINT('Ctrl Pts',(-0.305668184856449,0.104682534491432,
1.46687214536364));
#6689=CARTESIAN_POINT('Ctrl Pts',(-0.315820032591246,-0.0743007733969036,
1.48040059247731));
#6690=CARTESIAN_POINT('Ctrl Pts',(-0.250581817185145,-0.192431453073831,
1.49058865012208));
#6691=CARTESIAN_POINT('Ctrl Pts',(-0.184885616277594,-0.249388366415835,
1.49739790674125));
#6692=CARTESIAN_POINT('Ctrl Pts',(-0.148390241821198,-0.273082371347815,
1.50080595723938));
#6693=CARTESIAN_POINT('Ctrl Pts',(-0.108871032283292,-0.29139234917315,
1.50421741983629));
#6694=CARTESIAN_POINT('Ctrl Pts',(-0.0069453324122751,-0.322535646049005,
1.51256485573429));
#6695=CARTESIAN_POINT('Ctrl Pts',(0.173036139719135,-0.295879163364944,
1.52588654224678));
#6696=CARTESIAN_POINT('Ctrl Pts',(0.329381275573112,-0.0995231210697565,
1.54425036939462));
#6697=CARTESIAN_POINT('Ctrl Pts',(0.312519823715869,0.130664619012925,1.56116776183919));
#6698=CARTESIAN_POINT('Ctrl Pts',(0.175623409891217,0.283196568811908,1.57661184582646));
#6699=CARTESIAN_POINT('Ctrl Pts',(-0.00170640174969724,0.334465005486407,
1.59056005485894));
#6700=CARTESIAN_POINT('Ctrl Pts',(-0.180023541764348,0.283195393823563,
1.60455538622492));
#6701=CARTESIAN_POINT('Ctrl Pts',(-0.304003293840334,0.144546913461868,
1.61859632997908));
#6702=CARTESIAN_POINT('Ctrl Pts',(-0.335368767729676,-0.0394152680933303,
1.63268129545808));
#6703=CARTESIAN_POINT('Ctrl Pts',(-0.263809464751215,-0.212364713608931,
1.64680860320332));
#6704=CARTESIAN_POINT('Ctrl Pts',(-0.110777353802162,-0.321042679653587,
1.66097649136357));
#6705=CARTESIAN_POINT('Ctrl Pts',(0.0771377319574853,-0.331662145388596,
1.67518312328143));
#6706=CARTESIAN_POINT('Ctrl Pts',(0.242310499059917,-0.240422185372272,
1.68942658430208));
#6707=CARTESIAN_POINT('Ctrl Pts',(0.333965165875749,-0.0749639048060816,
1.70370489167579));
#6708=CARTESIAN_POINT('Ctrl Pts',(0.323334808639096,0.114391665751362,1.71801599173701));
#6709=CARTESIAN_POINT('Ctrl Pts',(0.213428807823085,0.269386973572793,1.73235777220482));
#6710=CARTESIAN_POINT('Ctrl Pts',(0.0375551957208218,0.342290293088701,
1.74672805867088));
#6711=CARTESIAN_POINT('Ctrl Pts',(-0.150552157108958,0.310435266995363,
1.76112462104241));
#6712=CARTESIAN_POINT('Ctrl Pts',(-0.292943546037226,0.183080826664645,
1.7755451807512));
#6713=CARTESIAN_POINT('Ctrl Pts',(-0.345971724616545,-0.000755050169826696,
1.78998741229651));
#6714=CARTESIAN_POINT('Ctrl Pts',(-0.292969625414991,-0.184869584225357,
1.80444894933381));
#6715=CARTESIAN_POINT('Ctrl Pts',(-0.149964130695888,-0.312702949838195,
1.81892738366057));
#6716=CARTESIAN_POINT('Ctrl Pts',(0.0393278383702601,-0.344893411306051,
1.83342028161105));
#6717=CARTESIAN_POINT('Ctrl Pts',(0.216880569645654,-0.271353329755712,
1.84792517694669));
#6718=CARTESIAN_POINT('Ctrl Pts',(0.32816306590606,-0.114557947655581,1.86243958044385));
#6719=CARTESIAN_POINT('Ctrl Pts',(0.338976565498085,0.077604733921516,1.87696098559129));
#6720=CARTESIAN_POINT('Ctrl Pts',(0.245857394029791,0.245901091257368,1.8914868739057));
#6721=CARTESIAN_POINT('Ctrl Pts',(0.0587650041824393,0.349754038023421,
1.90762891978624));
#6722=CARTESIAN_POINT('Ctrl Pts',(-0.181113967151586,0.314103429348402,
1.92538434383923));
#6723=CARTESIAN_POINT('Ctrl Pts',(-0.3457209249242,0.106820407791971,1.94474686926749));
#6724=CARTESIAN_POINT('Ctrl Pts',(-0.329429326627219,-0.112545408830404,
1.96087146849268));
#6725=CARTESIAN_POINT('Ctrl Pts',(-0.229624239431613,-0.246663510889421,
1.97376168226292));
#6726=CARTESIAN_POINT('Ctrl Pts',(-0.0883709022792632,-0.335964900532689,
1.98664460529397));
#6727=CARTESIAN_POINT('Ctrl Pts',(0.0650538569064664,-0.336061455964098,
1.99790631348129));
#6728=CARTESIAN_POINT('Ctrl Pts',(0.175154846512334,-0.280150232411291,
2.00754964965835));
#6729=CARTESIAN_POINT('Ctrl Pts',(0.240313024233827,-0.230169139256515,
2.01397587403001));
#6730=CARTESIAN_POINT('Ctrl Pts',(0.327278516892606,-0.113059531596934,
2.02521445394406));
#6731=CARTESIAN_POINT('Ctrl Pts',(0.344164783870684,0.104896799870906,2.04124691031968));
#6732=CARTESIAN_POINT('Ctrl Pts',(0.180057434020278,0.310325992459091,2.06044404323233));
#6733=CARTESIAN_POINT('Ctrl Pts',(-0.0568089689745267,0.345505318367412,
2.07799813231589));
#6734=CARTESIAN_POINT('Ctrl Pts',(-0.24141865243425,0.243028671458529,2.09391813720595));
#6735=CARTESIAN_POINT('Ctrl Pts',(-0.332978054716675,0.0773726024996246,
2.1082144881335));
#6736=CARTESIAN_POINT('Ctrl Pts',(-0.322327341410981,-0.111361257795146,
2.12247707319913));
#6737=CARTESIAN_POINT('Ctrl Pts',(-0.213201521733808,-0.265029708724835,
2.13670391728446));
#6738=CARTESIAN_POINT('Ctrl Pts',(-0.0395013579051905,-0.33691517309109,
2.15089294308459));
#6739=CARTESIAN_POINT('Ctrl Pts',(0.145288666887708,-0.305489063077451,
2.16504251556762));
#6740=CARTESIAN_POINT('Ctrl Pts',(0.284599775362727,-0.18083938172608,2.17915024381374));
#6741=CARTESIAN_POINT('Ctrl Pts',(0.318914082780001,-0.0616119635988021,
2.18852795857496));
#6742=CARTESIAN_POINT('Ctrl Pts',(0.318922161847072,-0.0018193816533177,
2.19320865445115));
#6743=CARTESIAN_POINT('',(0.299999683646987,0.00234130352927724,1.40009150124657));
#6744=CARTESIAN_POINT('Origin',(0.3,1.73141260914431E-17,1.43));
#6745=CARTESIAN_POINT('',(0.318922161847072,-0.00181938165331771,2.19320865445115));
#6746=CARTESIAN_POINT('Ctrl Pts',(0.299999683646987,0.00234130352927725,
1.40009150124657));
#6747=CARTESIAN_POINT('Ctrl Pts',(0.299992075807792,0.058646317336039,1.40449918252257));
#6748=CARTESIAN_POINT('Ctrl Pts',(0.267703823976176,0.170873854805974,1.41332597689034));
#6749=CARTESIAN_POINT('Ctrl Pts',(0.136388292868123,0.288427001435921,1.42662720914847));
#6750=CARTESIAN_POINT('Ctrl Pts',(-0.0380600582278086,0.318117946543192,
1.43998475699785));
#6751=CARTESIAN_POINT('Ctrl Pts',(-0.202303265104397,0.250195717548651,
1.45340015631867));
#6752=CARTESIAN_POINT('Ctrl Pts',(-0.305668184856449,0.104682534491432,
1.46687214536364));
#6753=CARTESIAN_POINT('Ctrl Pts',(-0.315820032591246,-0.0743007733969036,
1.48040059247731));
#6754=CARTESIAN_POINT('Ctrl Pts',(-0.250581817185145,-0.192431453073831,
1.49058865012208));
#6755=CARTESIAN_POINT('Ctrl Pts',(-0.184885616277594,-0.249388366415835,
1.49739790674125));
#6756=CARTESIAN_POINT('Ctrl Pts',(-0.148390241821198,-0.273082371347815,
1.50080595723938));
#6757=CARTESIAN_POINT('Ctrl Pts',(-0.108871032283292,-0.29139234917315,
1.50421741983629));
#6758=CARTESIAN_POINT('Ctrl Pts',(-0.0069453324122751,-0.322535646049005,
1.51256485573429));
#6759=CARTESIAN_POINT('Ctrl Pts',(0.173036139719135,-0.295879163364944,
1.52588654224678));
#6760=CARTESIAN_POINT('Ctrl Pts',(0.329381275573112,-0.0995231210697565,
1.54425036939462));
#6761=CARTESIAN_POINT('Ctrl Pts',(0.312519823715869,0.130664619012925,1.56116776183919));
#6762=CARTESIAN_POINT('Ctrl Pts',(0.175623409891217,0.283196568811908,1.57661184582646));
#6763=CARTESIAN_POINT('Ctrl Pts',(-0.00170640174969724,0.334465005486407,
1.59056005485894));
#6764=CARTESIAN_POINT('Ctrl Pts',(-0.180023541764348,0.283195393823563,
1.60455538622492));
#6765=CARTESIAN_POINT('Ctrl Pts',(-0.304003293840334,0.144546913461868,
1.61859632997908));
#6766=CARTESIAN_POINT('Ctrl Pts',(-0.335368767729676,-0.0394152680933303,
1.63268129545808));
#6767=CARTESIAN_POINT('Ctrl Pts',(-0.263809464751215,-0.212364713608931,
1.64680860320332));
#6768=CARTESIAN_POINT('Ctrl Pts',(-0.110777353802162,-0.321042679653587,
1.66097649136357));
#6769=CARTESIAN_POINT('Ctrl Pts',(0.0771377319574853,-0.331662145388596,
1.67518312328143));
#6770=CARTESIAN_POINT('Ctrl Pts',(0.242310499059917,-0.240422185372272,
1.68942658430208));
#6771=CARTESIAN_POINT('Ctrl Pts',(0.333965165875749,-0.0749639048060816,
1.70370489167579));
#6772=CARTESIAN_POINT('Ctrl Pts',(0.323334808639096,0.114391665751362,1.71801599173701));
#6773=CARTESIAN_POINT('Ctrl Pts',(0.213428807823085,0.269386973572793,1.73235777220482));
#6774=CARTESIAN_POINT('Ctrl Pts',(0.0375551957208218,0.342290293088701,
1.74672805867088));
#6775=CARTESIAN_POINT('Ctrl Pts',(-0.150552157108958,0.310435266995363,
1.76112462104241));
#6776=CARTESIAN_POINT('Ctrl Pts',(-0.292943546037226,0.183080826664645,
1.7755451807512));
#6777=CARTESIAN_POINT('Ctrl Pts',(-0.345971724616545,-0.000755050169826696,
1.78998741229651));
#6778=CARTESIAN_POINT('Ctrl Pts',(-0.292969625414991,-0.184869584225357,
1.80444894933381));
#6779=CARTESIAN_POINT('Ctrl Pts',(-0.149964130695888,-0.312702949838195,
1.81892738366057));
#6780=CARTESIAN_POINT('Ctrl Pts',(0.0393278383702601,-0.344893411306051,
1.83342028161105));
#6781=CARTESIAN_POINT('Ctrl Pts',(0.216880569645654,-0.271353329755712,
1.84792517694669));
#6782=CARTESIAN_POINT('Ctrl Pts',(0.32816306590606,-0.114557947655581,1.86243958044385));
#6783=CARTESIAN_POINT('Ctrl Pts',(0.338976565498085,0.077604733921516,1.87696098559129));
#6784=CARTESIAN_POINT('Ctrl Pts',(0.245857394029791,0.245901091257368,1.8914868739057));
#6785=CARTESIAN_POINT('Ctrl Pts',(0.0587650041824393,0.349754038023421,
1.90762891978624));
#6786=CARTESIAN_POINT('Ctrl Pts',(-0.181113967151586,0.314103429348402,
1.92538434383923));
#6787=CARTESIAN_POINT('Ctrl Pts',(-0.3457209249242,0.106820407791971,1.94474686926749));
#6788=CARTESIAN_POINT('Ctrl Pts',(-0.329429326627219,-0.112545408830404,
1.96087146849268));
#6789=CARTESIAN_POINT('Ctrl Pts',(-0.229624239431613,-0.246663510889421,
1.97376168226292));
#6790=CARTESIAN_POINT('Ctrl Pts',(-0.0883709022792632,-0.335964900532689,
1.98664460529397));
#6791=CARTESIAN_POINT('Ctrl Pts',(0.0650538569064664,-0.336061455964098,
1.99790631348129));
#6792=CARTESIAN_POINT('Ctrl Pts',(0.175154846512334,-0.280150232411291,
2.00754964965835));
#6793=CARTESIAN_POINT('Ctrl Pts',(0.240313024233827,-0.230169139256515,
2.01397587403001));
#6794=CARTESIAN_POINT('Ctrl Pts',(0.327278516892606,-0.113059531596934,
2.02521445394406));
#6795=CARTESIAN_POINT('Ctrl Pts',(0.344164783870684,0.104896799870906,2.04124691031968));
#6796=CARTESIAN_POINT('Ctrl Pts',(0.180057434020278,0.310325992459091,2.06044404323233));
#6797=CARTESIAN_POINT('Ctrl Pts',(-0.0568089689745267,0.345505318367412,
2.07799813231589));
#6798=CARTESIAN_POINT('Ctrl Pts',(-0.24141865243425,0.243028671458529,2.09391813720595));
#6799=CARTESIAN_POINT('Ctrl Pts',(-0.332978054716675,0.0773726024996246,
2.1082144881335));
#6800=CARTESIAN_POINT('Ctrl Pts',(-0.322327341410981,-0.111361257795146,
2.12247707319913));
#6801=CARTESIAN_POINT('Ctrl Pts',(-0.213201521733808,-0.265029708724835,
2.13670391728446));
#6802=CARTESIAN_POINT('Ctrl Pts',(-0.0395013579051905,-0.33691517309109,
2.15089294308459));
#6803=CARTESIAN_POINT('Ctrl Pts',(0.145288666887708,-0.305489063077451,
2.16504251556762));
#6804=CARTESIAN_POINT('Ctrl Pts',(0.284599775362727,-0.18083938172608,2.17915024381374));
#6805=CARTESIAN_POINT('Ctrl Pts',(0.318914082780001,-0.0616119635988021,
2.18852795857496));
#6806=CARTESIAN_POINT('Ctrl Pts',(0.318922161847072,-0.0018193816533177,
2.19320865445115));
#6807=CARTESIAN_POINT('Origin',(0.3,-3.60822483003176E-16,2.17));
#6808=CARTESIAN_POINT('Origin',(0.3,-3.60822483003176E-16,2.17));
#6809=CARTESIAN_POINT('Origin',(0.3,1.73141260914431E-17,1.43));
#8385=UNCERTAINTY_MEASURE_WITH_UNIT(LENGTH_MEASURE(0.001),#8429,
'DISTANCE_ACCURACY_VALUE',
'Maximum model space distance between geometric entities at asserted c
onnectivities');
#8402=UNCERTAINTY_MEASURE_WITH_UNIT(LENGTH_MEASURE(0.001),#8429,
'DISTANCE_ACCURACY_VALUE',
'Maximum model space distance between geometric entities at asserted c
onnectivities');
#8411=(
GEOMETRIC_REPRESENTATION_CONTEXT(3)
GLOBAL_UNCERTAINTY_ASSIGNED_CONTEXT((#8385))
GLOBAL_UNIT_ASSIGNED_CONTEXT((#8429,#8431,#8432))
REPRESENTATION_CONTEXT('','3D')
);
#8428=(
GEOMETRIC_REPRESENTATION_CONTEXT(3)
GLOBAL_UNCERTAINTY_ASSIGNED_CONTEXT((#8402))
GLOBAL_UNIT_ASSIGNED_CONTEXT((#8429,#8431,#8432))
REPRESENTATION_CONTEXT('','3D')
);
#8429=(
LENGTH_UNIT()
NAMED_UNIT(*)
SI_UNIT(.CENTI.,.METRE.)
);
#8431=(
NAMED_UNIT(*)
PLANE_ANGLE_UNIT()
SI_UNIT($,.RADIAN.)
);
#8432=(
NAMED_UNIT(*)
SI_UNIT($,.STERADIAN.)
SOLID_ANGLE_UNIT()
);
#8441=SHAPE_DEFINITION_REPRESENTATION(#8466,#8522);
#8466=PRODUCT_DEFINITION_SHAPE('',$,#8548);
#8522=SHAPE_REPRESENTATION('',(#4108),#8411);
#8539=PRODUCT_DEFINITION_CONTEXT('part definition',#8616,'design');
#8548=PRODUCT_DEFINITION('Poppet return spring',
'Poppet return spring',#8573,#8539);
#8573=PRODUCT_DEFINITION_FORMATION('',$,#8626);
#8616=APPLICATION_CONTEXT(
'Core Data for Automotive Mechanical Design Process');
#8617=PRODUCT_CONTEXT('part definition',#8616,'mechanical');
#8626=PRODUCT('Poppet return spring','Poppet return spring',
'Poppet return spring',(#8617));
#8699=COLOUR_RGB('Grey',0.48,0.52,0.57);
#8700=FILL_AREA_STYLE_COLOUR('',#8699);
#8701=FILL_AREA_STYLE('',(#8700));
#8702=SURFACE_STYLE_FILL_AREA(#8701);
#8703=SURFACE_SIDE_STYLE('',(#8702));
#8704=SURFACE_STYLE_USAGE(.BOTH.,#8703);
#8705=PRESENTATION_STYLE_ASSIGNMENT((#8704));
ENDSEC;
END-ISO-10303-21;
